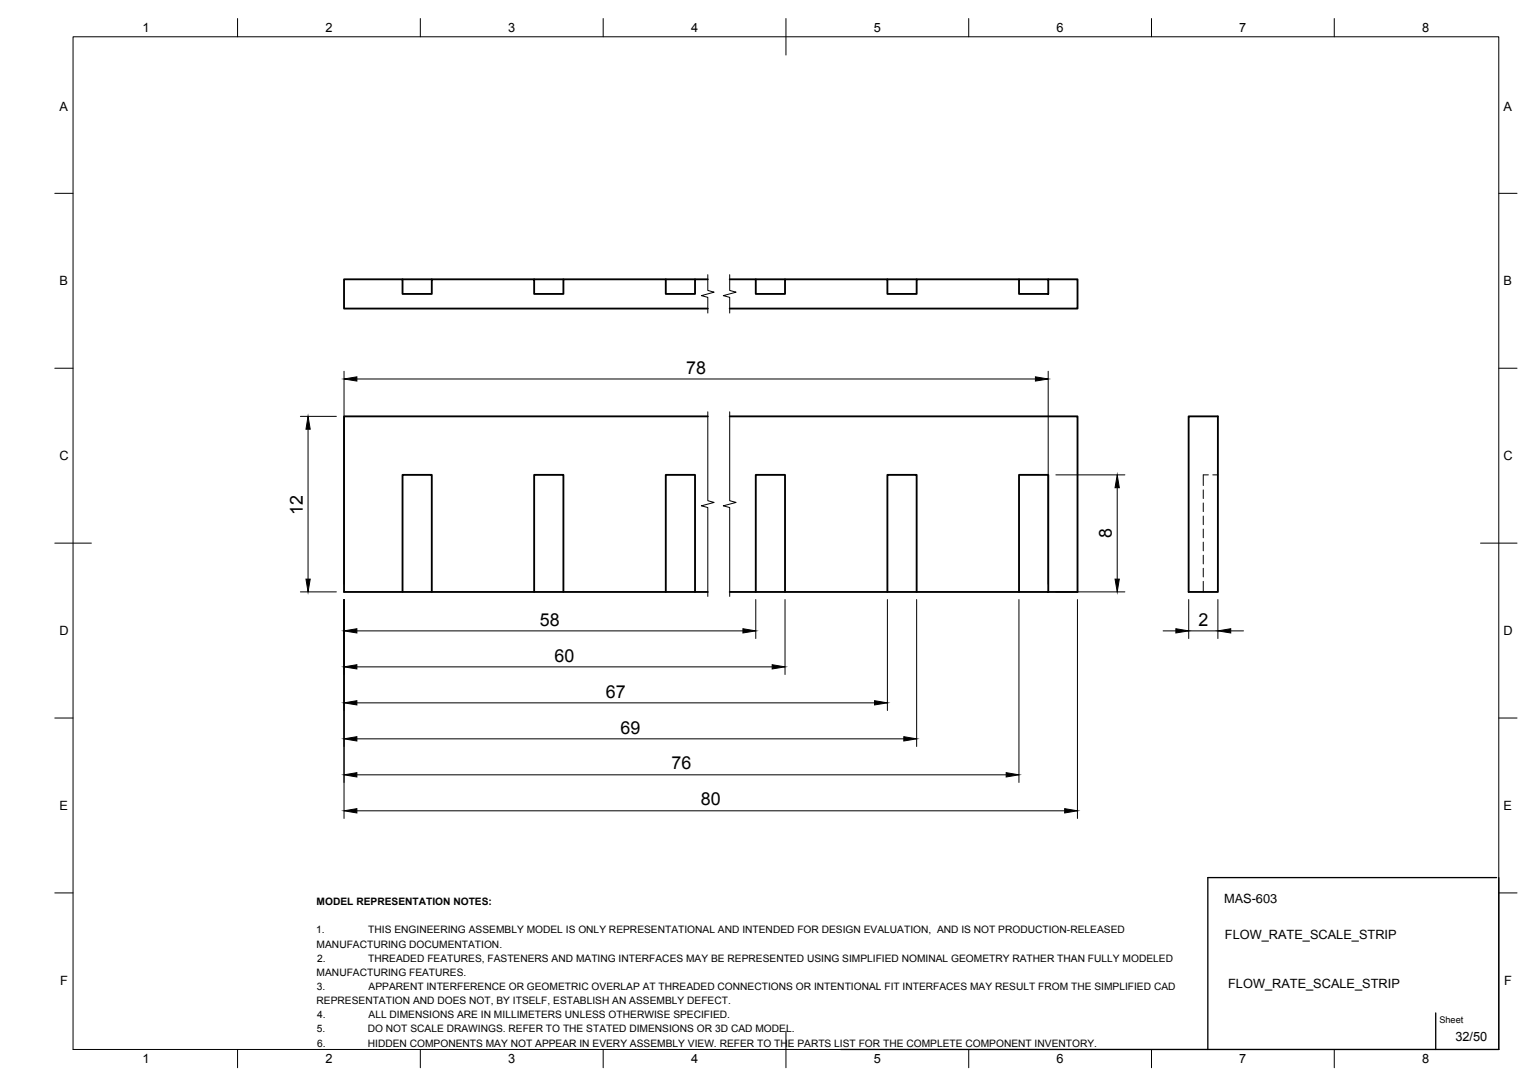
ISO-10303-21;
HEADER;
FILE_DESCRIPTION((''),'2;1');
FILE_NAME('FLOW_RATE_SCALE_STRIP.step','2026-10-01T22:06:14-07:00',(''),(''),'','','');
FILE_SCHEMA (('AUTOMOTIVE_DESIGN { 1 0 10303 214 3 1 1 }'));
ENDSEC;
DATA;
#10=MECHANICAL_DESIGN_GEOMETRIC_PRESENTATION_REPRESENTATION('',(#1004),#50440);
#912=SHAPE_REPRESENTATION_RELATIONSHIP('SRR','None',#50645,#957) ;
#957=ADVANCED_BREP_SHAPE_REPRESENTATION('',(#1059),#50414) ;
#1004=STYLED_ITEM('',(#50886),#1059) ;
#1059=MANIFOLD_SOLID_BREP('FLOW_RATE_SCALE_STRIP',#28671) ;
#2152=PLANE('',#30766) ;
#2153=PLANE('',#30767) ;
#2154=PLANE('',#30768) ;
#2155=PLANE('',#30769) ;
#2156=PLANE('',#30770) ;
#2157=PLANE('',#30771) ;
#2158=PLANE('',#30772) ;
#2159=PLANE('',#30773) ;
#2160=PLANE('',#30774) ;
#2161=PLANE('',#30775) ;
#2162=PLANE('',#30776) ;
#2163=PLANE('',#30777) ;
#2164=PLANE('',#30778) ;
#2165=PLANE('',#30779) ;
#2166=PLANE('',#30780) ;
#2167=PLANE('',#30781) ;
#2168=PLANE('',#30782) ;
#2169=PLANE('',#30783) ;
#2170=PLANE('',#30784) ;
#2171=PLANE('',#30785) ;
#2172=PLANE('',#30786) ;
#2173=PLANE('',#30787) ;
#2174=PLANE('',#30788) ;
#2175=PLANE('',#30789) ;
#2176=PLANE('',#30790) ;
#2177=PLANE('',#30791) ;
#2178=PLANE('',#30792) ;
#2179=PLANE('',#30793) ;
#2180=PLANE('',#30794) ;
#2181=PLANE('',#30795) ;
#2182=PLANE('',#30796) ;
#2183=PLANE('',#30797) ;
#2184=PLANE('',#30798) ;
#2185=PLANE('',#30799) ;
#2186=PLANE('',#30800) ;
#2187=PLANE('',#30801) ;
#2188=PLANE('',#30802) ;
#2189=PLANE('',#30803) ;
#2190=PLANE('',#30804) ;
#2191=PLANE('',#30805) ;
#2192=PLANE('',#30806) ;
#2193=PLANE('',#30807) ;
#3310=FACE_OUTER_BOUND('',#5090,.T.) ;
#3311=FACE_OUTER_BOUND('',#5091,.T.) ;
#3312=FACE_OUTER_BOUND('',#5092,.T.) ;
#3313=FACE_OUTER_BOUND('',#5093,.T.) ;
#3314=FACE_OUTER_BOUND('',#5094,.T.) ;
#3315=FACE_OUTER_BOUND('',#5095,.T.) ;
#3316=FACE_OUTER_BOUND('',#5096,.T.) ;
#3317=FACE_OUTER_BOUND('',#5097,.T.) ;
#3318=FACE_OUTER_BOUND('',#5098,.T.) ;
#3319=FACE_OUTER_BOUND('',#5099,.T.) ;
#3320=FACE_OUTER_BOUND('',#5100,.T.) ;
#3321=FACE_OUTER_BOUND('',#5101,.T.) ;
#3322=FACE_OUTER_BOUND('',#5102,.T.) ;
#3323=FACE_OUTER_BOUND('',#5103,.T.) ;
#3324=FACE_OUTER_BOUND('',#5104,.T.) ;
#3325=FACE_OUTER_BOUND('',#5105,.T.) ;
#3326=FACE_OUTER_BOUND('',#5106,.T.) ;
#3327=FACE_OUTER_BOUND('',#5107,.T.) ;
#3328=FACE_OUTER_BOUND('',#5108,.T.) ;
#3329=FACE_OUTER_BOUND('',#5109,.T.) ;
#3330=FACE_OUTER_BOUND('',#5110,.T.) ;
#3331=FACE_OUTER_BOUND('',#5111,.T.) ;
#3332=FACE_OUTER_BOUND('',#5112,.T.) ;
#3333=FACE_OUTER_BOUND('',#5113,.T.) ;
#3334=FACE_OUTER_BOUND('',#5114,.T.) ;
#3335=FACE_OUTER_BOUND('',#5115,.T.) ;
#3336=FACE_OUTER_BOUND('',#5116,.T.) ;
#3337=FACE_OUTER_BOUND('',#5117,.T.) ;
#3338=FACE_OUTER_BOUND('',#5118,.T.) ;
#3339=FACE_OUTER_BOUND('',#5119,.T.) ;
#3340=FACE_OUTER_BOUND('',#5120,.T.) ;
#3341=FACE_OUTER_BOUND('',#5121,.T.) ;
#3342=FACE_OUTER_BOUND('',#5122,.T.) ;
#3343=FACE_OUTER_BOUND('',#5123,.T.) ;
#3344=FACE_OUTER_BOUND('',#5124,.T.) ;
#3345=FACE_OUTER_BOUND('',#5125,.T.) ;
#3346=FACE_OUTER_BOUND('',#5126,.T.) ;
#3347=FACE_OUTER_BOUND('',#5127,.T.) ;
#3348=FACE_OUTER_BOUND('',#5128,.T.) ;
#3349=FACE_OUTER_BOUND('',#5129,.T.) ;
#3350=FACE_OUTER_BOUND('',#5130,.T.) ;
#3351=FACE_OUTER_BOUND('',#5131,.T.) ;
#5090=EDGE_LOOP('',(#23577,#23578,#23579,#23580)) ;
#5091=EDGE_LOOP('',(#23581,#23582,#23583,#23584)) ;
#5092=EDGE_LOOP('',(#23585,#23586,#23587,#23588)) ;
#5093=EDGE_LOOP('',(#23589,#23590,#23591,#23592)) ;
#5094=EDGE_LOOP('',(#23593,#23594,#23595,#23596,#23597,#23598,#23599,#23600,
#23601,#23602,#23603,#23604,#23605,#23606,#23607,#23608,#23609,#23610,#23611,
#23612,#23613,#23614,#23615,#23616,#23617,#23618,#23619,#23620,#23621,#23622,
#23623,#23624,#23625,#23626,#23627,#23628,#23629,#23630,#23631,#23632)) ;
#5095=EDGE_LOOP('',(#23633,#23634,#23635,#23636)) ;
#5096=EDGE_LOOP('',(#23637,#23638,#23639,#23640)) ;
#5097=EDGE_LOOP('',(#23641,#23642,#23643,#23644)) ;
#5098=EDGE_LOOP('',(#23645,#23646,#23647,#23648)) ;
#5099=EDGE_LOOP('',(#23649,#23650,#23651,#23652,#23653,#23654,#23655,#23656,
#23657,#23658,#23659,#23660,#23661,#23662,#23663,#23664,#23665,#23666,#23667,
#23668,#23669,#23670,#23671,#23672,#23673,#23674,#23675,#23676,#23677,#23678,
#23679,#23680,#23681,#23682,#23683,#23684,#23685,#23686,#23687,#23688)) ;
#5100=EDGE_LOOP('',(#23689,#23690,#23691,#23692)) ;
#5101=EDGE_LOOP('',(#23693,#23694,#23695,#23696)) ;
#5102=EDGE_LOOP('',(#23697,#23698,#23699,#23700)) ;
#5103=EDGE_LOOP('',(#23701,#23702,#23703,#23704)) ;
#5104=EDGE_LOOP('',(#23705,#23706,#23707,#23708)) ;
#5105=EDGE_LOOP('',(#23709,#23710,#23711,#23712)) ;
#5106=EDGE_LOOP('',(#23713,#23714,#23715,#23716)) ;
#5107=EDGE_LOOP('',(#23717,#23718,#23719,#23720)) ;
#5108=EDGE_LOOP('',(#23721,#23722,#23723,#23724)) ;
#5109=EDGE_LOOP('',(#23725,#23726,#23727,#23728)) ;
#5110=EDGE_LOOP('',(#23729,#23730,#23731,#23732)) ;
#5111=EDGE_LOOP('',(#23733,#23734,#23735,#23736)) ;
#5112=EDGE_LOOP('',(#23737,#23738,#23739,#23740)) ;
#5113=EDGE_LOOP('',(#23741,#23742,#23743,#23744)) ;
#5114=EDGE_LOOP('',(#23745,#23746,#23747,#23748)) ;
#5115=EDGE_LOOP('',(#23749,#23750,#23751,#23752)) ;
#5116=EDGE_LOOP('',(#23753,#23754,#23755,#23756)) ;
#5117=EDGE_LOOP('',(#23757,#23758,#23759,#23760)) ;
#5118=EDGE_LOOP('',(#23761,#23762,#23763,#23764)) ;
#5119=EDGE_LOOP('',(#23765,#23766,#23767,#23768)) ;
#5120=EDGE_LOOP('',(#23769,#23770,#23771,#23772)) ;
#5121=EDGE_LOOP('',(#23773,#23774,#23775,#23776)) ;
#5122=EDGE_LOOP('',(#23777,#23778,#23779,#23780)) ;
#5123=EDGE_LOOP('',(#23781,#23782,#23783,#23784)) ;
#5124=EDGE_LOOP('',(#23785,#23786,#23787,#23788)) ;
#5125=EDGE_LOOP('',(#23789,#23790,#23791,#23792)) ;
#5126=EDGE_LOOP('',(#23793,#23794,#23795,#23796)) ;
#5127=EDGE_LOOP('',(#23797,#23798,#23799,#23800)) ;
#5128=EDGE_LOOP('',(#23801,#23802,#23803,#23804)) ;
#5129=EDGE_LOOP('',(#23805,#23806,#23807,#23808)) ;
#5130=EDGE_LOOP('',(#23809,#23810,#23811,#23812)) ;
#5131=EDGE_LOOP('',(#23813,#23814,#23815,#23816)) ;
#7679=LINE('',#46561,#10151) ;
#7680=LINE('',#46563,#10152) ;
#7681=LINE('',#46565,#10153) ;
#7682=LINE('',#46566,#10154) ;
#7683=LINE('',#46569,#10155) ;
#7684=LINE('',#46571,#10156) ;
#7685=LINE('',#46572,#10157) ;
#7686=LINE('',#46575,#10158) ;
#7687=LINE('',#46576,#10159) ;
#7688=LINE('',#46579,#10160) ;
#7689=LINE('',#46580,#10161) ;
#7690=LINE('',#46583,#10162) ;
#7691=LINE('',#46585,#10163) ;
#7692=LINE('',#46587,#10164) ;
#7693=LINE('',#46589,#10165) ;
#7694=LINE('',#46591,#10166) ;
#7695=LINE('',#46593,#10167) ;
#7696=LINE('',#46595,#10168) ;
#7697=LINE('',#46597,#10169) ;
#7698=LINE('',#46599,#10170) ;
#7699=LINE('',#46601,#10171) ;
#7700=LINE('',#46603,#10172) ;
#7701=LINE('',#46605,#10173) ;
#7702=LINE('',#46607,#10174) ;
#7703=LINE('',#46609,#10175) ;
#7704=LINE('',#46611,#10176) ;
#7705=LINE('',#46613,#10177) ;
#7706=LINE('',#46615,#10178) ;
#7707=LINE('',#46617,#10179) ;
#7708=LINE('',#46619,#10180) ;
#7709=LINE('',#46621,#10181) ;
#7710=LINE('',#46623,#10182) ;
#7711=LINE('',#46625,#10183) ;
#7712=LINE('',#46627,#10184) ;
#7713=LINE('',#46629,#10185) ;
#7714=LINE('',#46631,#10186) ;
#7715=LINE('',#46633,#10187) ;
#7716=LINE('',#46635,#10188) ;
#7717=LINE('',#46637,#10189) ;
#7718=LINE('',#46639,#10190) ;
#7719=LINE('',#46641,#10191) ;
#7720=LINE('',#46643,#10192) ;
#7721=LINE('',#46645,#10193) ;
#7722=LINE('',#46647,#10194) ;
#7723=LINE('',#46649,#10195) ;
#7724=LINE('',#46651,#10196) ;
#7725=LINE('',#46653,#10197) ;
#7726=LINE('',#46654,#10198) ;
#7727=LINE('',#46658,#10199) ;
#7728=LINE('',#46660,#10200) ;
#7729=LINE('',#46662,#10201) ;
#7730=LINE('',#46663,#10202) ;
#7731=LINE('',#46665,#10203) ;
#7732=LINE('',#46666,#10204) ;
#7733=LINE('',#46668,#10205) ;
#7734=LINE('',#46670,#10206) ;
#7735=LINE('',#46673,#10207) ;
#7736=LINE('',#46675,#10208) ;
#7737=LINE('',#46676,#10209) ;
#7738=LINE('',#46678,#10210) ;
#7739=LINE('',#46680,#10211) ;
#7740=LINE('',#46681,#10212) ;
#7741=LINE('',#46683,#10213) ;
#7742=LINE('',#46685,#10214) ;
#7743=LINE('',#46686,#10215) ;
#7744=LINE('',#46688,#10216) ;
#7745=LINE('',#46690,#10217) ;
#7746=LINE('',#46691,#10218) ;
#7747=LINE('',#46693,#10219) ;
#7748=LINE('',#46695,#10220) ;
#7749=LINE('',#46696,#10221) ;
#7750=LINE('',#46698,#10222) ;
#7751=LINE('',#46700,#10223) ;
#7752=LINE('',#46701,#10224) ;
#7753=LINE('',#46703,#10225) ;
#7754=LINE('',#46705,#10226) ;
#7755=LINE('',#46706,#10227) ;
#7756=LINE('',#46708,#10228) ;
#7757=LINE('',#46710,#10229) ;
#7758=LINE('',#46711,#10230) ;
#7759=LINE('',#46714,#10231) ;
#7760=LINE('',#46716,#10232) ;
#7761=LINE('',#46717,#10233) ;
#7762=LINE('',#46719,#10234) ;
#7763=LINE('',#46721,#10235) ;
#7764=LINE('',#46725,#10236) ;
#7765=LINE('',#46727,#10237) ;
#7766=LINE('',#46728,#10238) ;
#7767=LINE('',#46730,#10239) ;
#7768=LINE('',#46732,#10240) ;
#7769=LINE('',#46736,#10241) ;
#7770=LINE('',#46738,#10242) ;
#7771=LINE('',#46739,#10243) ;
#7772=LINE('',#46741,#10244) ;
#7773=LINE('',#46743,#10245) ;
#7774=LINE('',#46747,#10246) ;
#7775=LINE('',#46749,#10247) ;
#7776=LINE('',#46750,#10248) ;
#7777=LINE('',#46752,#10249) ;
#7778=LINE('',#46754,#10250) ;
#7779=LINE('',#46758,#10251) ;
#7780=LINE('',#46760,#10252) ;
#7781=LINE('',#46761,#10253) ;
#7782=LINE('',#46763,#10254) ;
#7783=LINE('',#46765,#10255) ;
#7784=LINE('',#46769,#10256) ;
#7785=LINE('',#46771,#10257) ;
#7786=LINE('',#46772,#10258) ;
#7787=LINE('',#46774,#10259) ;
#7788=LINE('',#46776,#10260) ;
#7789=LINE('',#46780,#10261) ;
#7790=LINE('',#46782,#10262) ;
#7791=LINE('',#46783,#10263) ;
#7792=LINE('',#46785,#10264) ;
#7793=LINE('',#46787,#10265) ;
#7794=LINE('',#46791,#10266) ;
#7795=LINE('',#46793,#10267) ;
#7796=LINE('',#46794,#10268) ;
#7797=LINE('',#46796,#10269) ;
#7798=LINE('',#46798,#10270) ;
#10151=VECTOR('',#37438,1.) ;
#10152=VECTOR('',#37439,1.) ;
#10153=VECTOR('',#37440,1.) ;
#10154=VECTOR('',#37441,1.) ;
#10155=VECTOR('',#37444,1.) ;
#10156=VECTOR('',#37445,1.) ;
#10157=VECTOR('',#37446,1.) ;
#10158=VECTOR('',#37449,1.) ;
#10159=VECTOR('',#37450,1.) ;
#10160=VECTOR('',#37453,1.) ;
#10161=VECTOR('',#37454,1.) ;
#10162=VECTOR('',#37457,1.) ;
#10163=VECTOR('',#37458,1.) ;
#10164=VECTOR('',#37459,1.) ;
#10165=VECTOR('',#37460,1.) ;
#10166=VECTOR('',#37461,1.) ;
#10167=VECTOR('',#37462,1.) ;
#10168=VECTOR('',#37463,1.) ;
#10169=VECTOR('',#37464,1.) ;
#10170=VECTOR('',#37465,1.) ;
#10171=VECTOR('',#37466,1.) ;
#10172=VECTOR('',#37467,1.) ;
#10173=VECTOR('',#37468,1.) ;
#10174=VECTOR('',#37469,1.) ;
#10175=VECTOR('',#37470,1.) ;
#10176=VECTOR('',#37471,1.) ;
#10177=VECTOR('',#37472,1.) ;
#10178=VECTOR('',#37473,1.) ;
#10179=VECTOR('',#37474,1.) ;
#10180=VECTOR('',#37475,1.) ;
#10181=VECTOR('',#37476,1.) ;
#10182=VECTOR('',#37477,1.) ;
#10183=VECTOR('',#37478,1.) ;
#10184=VECTOR('',#37479,1.) ;
#10185=VECTOR('',#37480,1.) ;
#10186=VECTOR('',#37481,1.) ;
#10187=VECTOR('',#37482,1.) ;
#10188=VECTOR('',#37483,1.) ;
#10189=VECTOR('',#37484,1.) ;
#10190=VECTOR('',#37485,1.) ;
#10191=VECTOR('',#37486,1.) ;
#10192=VECTOR('',#37487,1.) ;
#10193=VECTOR('',#37488,1.) ;
#10194=VECTOR('',#37489,1.) ;
#10195=VECTOR('',#37490,1.) ;
#10196=VECTOR('',#37491,1.) ;
#10197=VECTOR('',#37492,1.) ;
#10198=VECTOR('',#37493,1.) ;
#10199=VECTOR('',#37496,1.) ;
#10200=VECTOR('',#37497,1.) ;
#10201=VECTOR('',#37498,1.) ;
#10202=VECTOR('',#37499,1.) ;
#10203=VECTOR('',#37502,1.) ;
#10204=VECTOR('',#37503,1.) ;
#10205=VECTOR('',#37506,1.) ;
#10206=VECTOR('',#37509,1.) ;
#10207=VECTOR('',#37512,1.) ;
#10208=VECTOR('',#37513,1.) ;
#10209=VECTOR('',#37514,1.) ;
#10210=VECTOR('',#37515,1.) ;
#10211=VECTOR('',#37516,1.) ;
#10212=VECTOR('',#37517,1.) ;
#10213=VECTOR('',#37518,1.) ;
#10214=VECTOR('',#37519,1.) ;
#10215=VECTOR('',#37520,1.) ;
#10216=VECTOR('',#37521,1.) ;
#10217=VECTOR('',#37522,1.) ;
#10218=VECTOR('',#37523,1.) ;
#10219=VECTOR('',#37524,1.) ;
#10220=VECTOR('',#37525,1.) ;
#10221=VECTOR('',#37526,1.) ;
#10222=VECTOR('',#37527,1.) ;
#10223=VECTOR('',#37528,1.) ;
#10224=VECTOR('',#37529,1.) ;
#10225=VECTOR('',#37530,1.) ;
#10226=VECTOR('',#37531,1.) ;
#10227=VECTOR('',#37532,1.) ;
#10228=VECTOR('',#37533,1.) ;
#10229=VECTOR('',#37534,1.) ;
#10230=VECTOR('',#37535,1.) ;
#10231=VECTOR('',#37538,1.) ;
#10232=VECTOR('',#37539,1.) ;
#10233=VECTOR('',#37540,1.) ;
#10234=VECTOR('',#37543,1.) ;
#10235=VECTOR('',#37546,1.) ;
#10236=VECTOR('',#37551,1.) ;
#10237=VECTOR('',#37552,1.) ;
#10238=VECTOR('',#37553,1.) ;
#10239=VECTOR('',#37556,1.) ;
#10240=VECTOR('',#37559,1.) ;
#10241=VECTOR('',#37564,1.) ;
#10242=VECTOR('',#37565,1.) ;
#10243=VECTOR('',#37566,1.) ;
#10244=VECTOR('',#37569,1.) ;
#10245=VECTOR('',#37572,1.) ;
#10246=VECTOR('',#37577,1.) ;
#10247=VECTOR('',#37578,1.) ;
#10248=VECTOR('',#37579,1.) ;
#10249=VECTOR('',#37582,1.) ;
#10250=VECTOR('',#37585,1.) ;
#10251=VECTOR('',#37590,1.) ;
#10252=VECTOR('',#37591,1.) ;
#10253=VECTOR('',#37592,1.) ;
#10254=VECTOR('',#37595,1.) ;
#10255=VECTOR('',#37598,1.) ;
#10256=VECTOR('',#37603,1.) ;
#10257=VECTOR('',#37604,1.) ;
#10258=VECTOR('',#37605,1.) ;
#10259=VECTOR('',#37608,1.) ;
#10260=VECTOR('',#37611,1.) ;
#10261=VECTOR('',#37616,1.) ;
#10262=VECTOR('',#37617,1.) ;
#10263=VECTOR('',#37618,1.) ;
#10264=VECTOR('',#37621,1.) ;
#10265=VECTOR('',#37624,1.) ;
#10266=VECTOR('',#37629,1.) ;
#10267=VECTOR('',#37630,1.) ;
#10268=VECTOR('',#37631,1.) ;
#10269=VECTOR('',#37634,1.) ;
#10270=VECTOR('',#37637,1.) ;
#13508=VERTEX_POINT('',#46559) ;
#13509=VERTEX_POINT('',#46560) ;
#13510=VERTEX_POINT('',#46562) ;
#13511=VERTEX_POINT('',#46564) ;
#13512=VERTEX_POINT('',#46568) ;
#13513=VERTEX_POINT('',#46570) ;
#13514=VERTEX_POINT('',#46574) ;
#13515=VERTEX_POINT('',#46578) ;
#13516=VERTEX_POINT('',#46582) ;
#13517=VERTEX_POINT('',#46584) ;
#13518=VERTEX_POINT('',#46586) ;
#13519=VERTEX_POINT('',#46588) ;
#13520=VERTEX_POINT('',#46590) ;
#13521=VERTEX_POINT('',#46592) ;
#13522=VERTEX_POINT('',#46594) ;
#13523=VERTEX_POINT('',#46596) ;
#13524=VERTEX_POINT('',#46598) ;
#13525=VERTEX_POINT('',#46600) ;
#13526=VERTEX_POINT('',#46602) ;
#13527=VERTEX_POINT('',#46604) ;
#13528=VERTEX_POINT('',#46606) ;
#13529=VERTEX_POINT('',#46608) ;
#13530=VERTEX_POINT('',#46610) ;
#13531=VERTEX_POINT('',#46612) ;
#13532=VERTEX_POINT('',#46614) ;
#13533=VERTEX_POINT('',#46616) ;
#13534=VERTEX_POINT('',#46618) ;
#13535=VERTEX_POINT('',#46620) ;
#13536=VERTEX_POINT('',#46622) ;
#13537=VERTEX_POINT('',#46624) ;
#13538=VERTEX_POINT('',#46626) ;
#13539=VERTEX_POINT('',#46628) ;
#13540=VERTEX_POINT('',#46630) ;
#13541=VERTEX_POINT('',#46632) ;
#13542=VERTEX_POINT('',#46634) ;
#13543=VERTEX_POINT('',#46636) ;
#13544=VERTEX_POINT('',#46638) ;
#13545=VERTEX_POINT('',#46640) ;
#13546=VERTEX_POINT('',#46642) ;
#13547=VERTEX_POINT('',#46644) ;
#13548=VERTEX_POINT('',#46646) ;
#13549=VERTEX_POINT('',#46648) ;
#13550=VERTEX_POINT('',#46650) ;
#13551=VERTEX_POINT('',#46652) ;
#13552=VERTEX_POINT('',#46656) ;
#13553=VERTEX_POINT('',#46657) ;
#13554=VERTEX_POINT('',#46659) ;
#13555=VERTEX_POINT('',#46661) ;
#13556=VERTEX_POINT('',#46672) ;
#13557=VERTEX_POINT('',#46674) ;
#13558=VERTEX_POINT('',#46677) ;
#13559=VERTEX_POINT('',#46679) ;
#13560=VERTEX_POINT('',#46682) ;
#13561=VERTEX_POINT('',#46684) ;
#13562=VERTEX_POINT('',#46687) ;
#13563=VERTEX_POINT('',#46689) ;
#13564=VERTEX_POINT('',#46692) ;
#13565=VERTEX_POINT('',#46694) ;
#13566=VERTEX_POINT('',#46697) ;
#13567=VERTEX_POINT('',#46699) ;
#13568=VERTEX_POINT('',#46702) ;
#13569=VERTEX_POINT('',#46704) ;
#13570=VERTEX_POINT('',#46707) ;
#13571=VERTEX_POINT('',#46709) ;
#13572=VERTEX_POINT('',#46713) ;
#13573=VERTEX_POINT('',#46715) ;
#13574=VERTEX_POINT('',#46724) ;
#13575=VERTEX_POINT('',#46726) ;
#13576=VERTEX_POINT('',#46735) ;
#13577=VERTEX_POINT('',#46737) ;
#13578=VERTEX_POINT('',#46746) ;
#13579=VERTEX_POINT('',#46748) ;
#13580=VERTEX_POINT('',#46757) ;
#13581=VERTEX_POINT('',#46759) ;
#13582=VERTEX_POINT('',#46768) ;
#13583=VERTEX_POINT('',#46770) ;
#13584=VERTEX_POINT('',#46779) ;
#13585=VERTEX_POINT('',#46781) ;
#13586=VERTEX_POINT('',#46790) ;
#13587=VERTEX_POINT('',#46792) ;
#17054=EDGE_CURVE('',#13508,#13509,#7679,.T.) ;
#17055=EDGE_CURVE('',#13510,#13508,#7680,.T.) ;
#17056=EDGE_CURVE('',#13511,#13510,#7681,.T.) ;
#17057=EDGE_CURVE('',#13509,#13511,#7682,.T.) ;
#17058=EDGE_CURVE('',#13509,#13512,#7683,.T.) ;
#17059=EDGE_CURVE('',#13513,#13511,#7684,.T.) ;
#17060=EDGE_CURVE('',#13512,#13513,#7685,.T.) ;
#17061=EDGE_CURVE('',#13513,#13514,#7686,.T.) ;
#17062=EDGE_CURVE('',#13514,#13510,#7687,.T.) ;
#17063=EDGE_CURVE('',#13515,#13508,#7688,.T.) ;
#17064=EDGE_CURVE('',#13514,#13515,#7689,.T.) ;
#17065=EDGE_CURVE('',#13516,#13512,#7690,.T.) ;
#17066=EDGE_CURVE('',#13516,#13517,#7691,.T.) ;
#17067=EDGE_CURVE('',#13517,#13518,#7692,.T.) ;
#17068=EDGE_CURVE('',#13518,#13519,#7693,.T.) ;
#17069=EDGE_CURVE('',#13520,#13519,#7694,.T.) ;
#17070=EDGE_CURVE('',#13520,#13521,#7695,.T.) ;
#17071=EDGE_CURVE('',#13521,#13522,#7696,.T.) ;
#17072=EDGE_CURVE('',#13522,#13523,#7697,.T.) ;
#17073=EDGE_CURVE('',#13524,#13523,#7698,.T.) ;
#17074=EDGE_CURVE('',#13524,#13525,#7699,.T.) ;
#17075=EDGE_CURVE('',#13525,#13526,#7700,.T.) ;
#17076=EDGE_CURVE('',#13526,#13527,#7701,.T.) ;
#17077=EDGE_CURVE('',#13528,#13527,#7702,.T.) ;
#17078=EDGE_CURVE('',#13528,#13529,#7703,.T.) ;
#17079=EDGE_CURVE('',#13529,#13530,#7704,.T.) ;
#17080=EDGE_CURVE('',#13530,#13531,#7705,.T.) ;
#17081=EDGE_CURVE('',#13532,#13531,#7706,.T.) ;
#17082=EDGE_CURVE('',#13532,#13533,#7707,.T.) ;
#17083=EDGE_CURVE('',#13533,#13534,#7708,.T.) ;
#17084=EDGE_CURVE('',#13534,#13535,#7709,.T.) ;
#17085=EDGE_CURVE('',#13536,#13535,#7710,.T.) ;
#17086=EDGE_CURVE('',#13536,#13537,#7711,.T.) ;
#17087=EDGE_CURVE('',#13537,#13538,#7712,.T.) ;
#17088=EDGE_CURVE('',#13538,#13539,#7713,.T.) ;
#17089=EDGE_CURVE('',#13540,#13539,#7714,.T.) ;
#17090=EDGE_CURVE('',#13540,#13541,#7715,.T.) ;
#17091=EDGE_CURVE('',#13541,#13542,#7716,.T.) ;
#17092=EDGE_CURVE('',#13542,#13543,#7717,.T.) ;
#17093=EDGE_CURVE('',#13544,#13543,#7718,.T.) ;
#17094=EDGE_CURVE('',#13544,#13545,#7719,.T.) ;
#17095=EDGE_CURVE('',#13545,#13546,#7720,.T.) ;
#17096=EDGE_CURVE('',#13546,#13547,#7721,.T.) ;
#17097=EDGE_CURVE('',#13548,#13547,#7722,.T.) ;
#17098=EDGE_CURVE('',#13548,#13549,#7723,.T.) ;
#17099=EDGE_CURVE('',#13550,#13549,#7724,.T.) ;
#17100=EDGE_CURVE('',#13551,#13550,#7725,.T.) ;
#17101=EDGE_CURVE('',#13515,#13551,#7726,.T.) ;
#17102=EDGE_CURVE('',#13552,#13553,#7727,.T.) ;
#17103=EDGE_CURVE('',#13552,#13554,#7728,.T.) ;
#17104=EDGE_CURVE('',#13554,#13555,#7729,.T.) ;
#17105=EDGE_CURVE('',#13553,#13555,#7730,.T.) ;
#17106=EDGE_CURVE('',#13553,#13516,#7731,.T.) ;
#17107=EDGE_CURVE('',#13555,#13517,#7732,.T.) ;
#17108=EDGE_CURVE('',#13518,#13554,#7733,.T.) ;
#17109=EDGE_CURVE('',#13519,#13552,#7734,.T.) ;
#17110=EDGE_CURVE('',#13551,#13556,#7735,.T.) ;
#17111=EDGE_CURVE('',#13556,#13557,#7736,.T.) ;
#17112=EDGE_CURVE('',#13557,#13548,#7737,.T.) ;
#17113=EDGE_CURVE('',#13547,#13558,#7738,.T.) ;
#17114=EDGE_CURVE('',#13558,#13559,#7739,.T.) ;
#17115=EDGE_CURVE('',#13559,#13544,#7740,.T.) ;
#17116=EDGE_CURVE('',#13543,#13560,#7741,.T.) ;
#17117=EDGE_CURVE('',#13560,#13561,#7742,.T.) ;
#17118=EDGE_CURVE('',#13561,#13540,#7743,.T.) ;
#17119=EDGE_CURVE('',#13539,#13562,#7744,.T.) ;
#17120=EDGE_CURVE('',#13562,#13563,#7745,.T.) ;
#17121=EDGE_CURVE('',#13563,#13536,#7746,.T.) ;
#17122=EDGE_CURVE('',#13535,#13564,#7747,.T.) ;
#17123=EDGE_CURVE('',#13564,#13565,#7748,.T.) ;
#17124=EDGE_CURVE('',#13565,#13532,#7749,.T.) ;
#17125=EDGE_CURVE('',#13531,#13566,#7750,.T.) ;
#17126=EDGE_CURVE('',#13566,#13567,#7751,.T.) ;
#17127=EDGE_CURVE('',#13567,#13528,#7752,.T.) ;
#17128=EDGE_CURVE('',#13527,#13568,#7753,.T.) ;
#17129=EDGE_CURVE('',#13568,#13569,#7754,.T.) ;
#17130=EDGE_CURVE('',#13569,#13524,#7755,.T.) ;
#17131=EDGE_CURVE('',#13523,#13570,#7756,.T.) ;
#17132=EDGE_CURVE('',#13570,#13571,#7757,.T.) ;
#17133=EDGE_CURVE('',#13571,#13520,#7758,.T.) ;
#17134=EDGE_CURVE('',#13572,#13521,#7759,.T.) ;
#17135=EDGE_CURVE('',#13573,#13572,#7760,.T.) ;
#17136=EDGE_CURVE('',#13522,#13573,#7761,.T.) ;
#17137=EDGE_CURVE('',#13570,#13573,#7762,.T.) ;
#17138=EDGE_CURVE('',#13571,#13572,#7763,.T.) ;
#17139=EDGE_CURVE('',#13568,#13574,#7764,.T.) ;
#17140=EDGE_CURVE('',#13574,#13575,#7765,.T.) ;
#17141=EDGE_CURVE('',#13569,#13575,#7766,.T.) ;
#17142=EDGE_CURVE('',#13575,#13525,#7767,.T.) ;
#17143=EDGE_CURVE('',#13526,#13574,#7768,.T.) ;
#17144=EDGE_CURVE('',#13576,#13529,#7769,.T.) ;
#17145=EDGE_CURVE('',#13577,#13576,#7770,.T.) ;
#17146=EDGE_CURVE('',#13530,#13577,#7771,.T.) ;
#17147=EDGE_CURVE('',#13566,#13577,#7772,.T.) ;
#17148=EDGE_CURVE('',#13567,#13576,#7773,.T.) ;
#17149=EDGE_CURVE('',#13564,#13578,#7774,.T.) ;
#17150=EDGE_CURVE('',#13578,#13579,#7775,.T.) ;
#17151=EDGE_CURVE('',#13565,#13579,#7776,.T.) ;
#17152=EDGE_CURVE('',#13579,#13533,#7777,.T.) ;
#17153=EDGE_CURVE('',#13534,#13578,#7778,.T.) ;
#17154=EDGE_CURVE('',#13580,#13537,#7779,.T.) ;
#17155=EDGE_CURVE('',#13581,#13580,#7780,.T.) ;
#17156=EDGE_CURVE('',#13538,#13581,#7781,.T.) ;
#17157=EDGE_CURVE('',#13562,#13581,#7782,.T.) ;
#17158=EDGE_CURVE('',#13563,#13580,#7783,.T.) ;
#17159=EDGE_CURVE('',#13560,#13582,#7784,.T.) ;
#17160=EDGE_CURVE('',#13582,#13583,#7785,.T.) ;
#17161=EDGE_CURVE('',#13561,#13583,#7786,.T.) ;
#17162=EDGE_CURVE('',#13583,#13541,#7787,.T.) ;
#17163=EDGE_CURVE('',#13542,#13582,#7788,.T.) ;
#17164=EDGE_CURVE('',#13584,#13545,#7789,.T.) ;
#17165=EDGE_CURVE('',#13585,#13584,#7790,.T.) ;
#17166=EDGE_CURVE('',#13546,#13585,#7791,.T.) ;
#17167=EDGE_CURVE('',#13558,#13585,#7792,.T.) ;
#17168=EDGE_CURVE('',#13559,#13584,#7793,.T.) ;
#17169=EDGE_CURVE('',#13586,#13550,#7794,.T.) ;
#17170=EDGE_CURVE('',#13549,#13587,#7795,.T.) ;
#17171=EDGE_CURVE('',#13587,#13586,#7796,.T.) ;
#17172=EDGE_CURVE('',#13557,#13587,#7797,.T.) ;
#17173=EDGE_CURVE('',#13556,#13586,#7798,.T.) ;
#23577=ORIENTED_EDGE('',*,*,#17054,.F.) ;
#23578=ORIENTED_EDGE('',*,*,#17055,.F.) ;
#23579=ORIENTED_EDGE('',*,*,#17056,.F.) ;
#23580=ORIENTED_EDGE('',*,*,#17057,.F.) ;
#23581=ORIENTED_EDGE('',*,*,#17058,.F.) ;
#23582=ORIENTED_EDGE('',*,*,#17057,.T.) ;
#23583=ORIENTED_EDGE('',*,*,#17059,.F.) ;
#23584=ORIENTED_EDGE('',*,*,#17060,.F.) ;
#23585=ORIENTED_EDGE('',*,*,#17061,.F.) ;
#23586=ORIENTED_EDGE('',*,*,#17059,.T.) ;
#23587=ORIENTED_EDGE('',*,*,#17056,.T.) ;
#23588=ORIENTED_EDGE('',*,*,#17062,.F.) ;
#23589=ORIENTED_EDGE('',*,*,#17063,.F.) ;
#23590=ORIENTED_EDGE('',*,*,#17064,.F.) ;
#23591=ORIENTED_EDGE('',*,*,#17062,.T.) ;
#23592=ORIENTED_EDGE('',*,*,#17055,.T.) ;
#23593=ORIENTED_EDGE('',*,*,#17063,.T.) ;
#23594=ORIENTED_EDGE('',*,*,#17054,.T.) ;
#23595=ORIENTED_EDGE('',*,*,#17058,.T.) ;
#23596=ORIENTED_EDGE('',*,*,#17065,.F.) ;
#23597=ORIENTED_EDGE('',*,*,#17066,.T.) ;
#23598=ORIENTED_EDGE('',*,*,#17067,.T.) ;
#23599=ORIENTED_EDGE('',*,*,#17068,.T.) ;
#23600=ORIENTED_EDGE('',*,*,#17069,.F.) ;
#23601=ORIENTED_EDGE('',*,*,#17070,.T.) ;
#23602=ORIENTED_EDGE('',*,*,#17071,.T.) ;
#23603=ORIENTED_EDGE('',*,*,#17072,.T.) ;
#23604=ORIENTED_EDGE('',*,*,#17073,.F.) ;
#23605=ORIENTED_EDGE('',*,*,#17074,.T.) ;
#23606=ORIENTED_EDGE('',*,*,#17075,.T.) ;
#23607=ORIENTED_EDGE('',*,*,#17076,.T.) ;
#23608=ORIENTED_EDGE('',*,*,#17077,.F.) ;
#23609=ORIENTED_EDGE('',*,*,#17078,.T.) ;
#23610=ORIENTED_EDGE('',*,*,#17079,.T.) ;
#23611=ORIENTED_EDGE('',*,*,#17080,.T.) ;
#23612=ORIENTED_EDGE('',*,*,#17081,.F.) ;
#23613=ORIENTED_EDGE('',*,*,#17082,.T.) ;
#23614=ORIENTED_EDGE('',*,*,#17083,.T.) ;
#23615=ORIENTED_EDGE('',*,*,#17084,.T.) ;
#23616=ORIENTED_EDGE('',*,*,#17085,.F.) ;
#23617=ORIENTED_EDGE('',*,*,#17086,.T.) ;
#23618=ORIENTED_EDGE('',*,*,#17087,.T.) ;
#23619=ORIENTED_EDGE('',*,*,#17088,.T.) ;
#23620=ORIENTED_EDGE('',*,*,#17089,.F.) ;
#23621=ORIENTED_EDGE('',*,*,#17090,.T.) ;
#23622=ORIENTED_EDGE('',*,*,#17091,.T.) ;
#23623=ORIENTED_EDGE('',*,*,#17092,.T.) ;
#23624=ORIENTED_EDGE('',*,*,#17093,.F.) ;
#23625=ORIENTED_EDGE('',*,*,#17094,.T.) ;
#23626=ORIENTED_EDGE('',*,*,#17095,.T.) ;
#23627=ORIENTED_EDGE('',*,*,#17096,.T.) ;
#23628=ORIENTED_EDGE('',*,*,#17097,.F.) ;
#23629=ORIENTED_EDGE('',*,*,#17098,.T.) ;
#23630=ORIENTED_EDGE('',*,*,#17099,.F.) ;
#23631=ORIENTED_EDGE('',*,*,#17100,.F.) ;
#23632=ORIENTED_EDGE('',*,*,#17101,.F.) ;
#23633=ORIENTED_EDGE('',*,*,#17102,.F.) ;
#23634=ORIENTED_EDGE('',*,*,#17103,.T.) ;
#23635=ORIENTED_EDGE('',*,*,#17104,.T.) ;
#23636=ORIENTED_EDGE('',*,*,#17105,.F.) ;
#23637=ORIENTED_EDGE('',*,*,#17106,.F.) ;
#23638=ORIENTED_EDGE('',*,*,#17105,.T.) ;
#23639=ORIENTED_EDGE('',*,*,#17107,.T.) ;
#23640=ORIENTED_EDGE('',*,*,#17066,.F.) ;
#23641=ORIENTED_EDGE('',*,*,#17067,.F.) ;
#23642=ORIENTED_EDGE('',*,*,#17107,.F.) ;
#23643=ORIENTED_EDGE('',*,*,#17104,.F.) ;
#23644=ORIENTED_EDGE('',*,*,#17108,.F.) ;
#23645=ORIENTED_EDGE('',*,*,#17109,.F.) ;
#23646=ORIENTED_EDGE('',*,*,#17068,.F.) ;
#23647=ORIENTED_EDGE('',*,*,#17108,.T.) ;
#23648=ORIENTED_EDGE('',*,*,#17103,.F.) ;
#23649=ORIENTED_EDGE('',*,*,#17064,.T.) ;
#23650=ORIENTED_EDGE('',*,*,#17101,.T.) ;
#23651=ORIENTED_EDGE('',*,*,#17110,.T.) ;
#23652=ORIENTED_EDGE('',*,*,#17111,.T.) ;
#23653=ORIENTED_EDGE('',*,*,#17112,.T.) ;
#23654=ORIENTED_EDGE('',*,*,#17097,.T.) ;
#23655=ORIENTED_EDGE('',*,*,#17113,.T.) ;
#23656=ORIENTED_EDGE('',*,*,#17114,.T.) ;
#23657=ORIENTED_EDGE('',*,*,#17115,.T.) ;
#23658=ORIENTED_EDGE('',*,*,#17093,.T.) ;
#23659=ORIENTED_EDGE('',*,*,#17116,.T.) ;
#23660=ORIENTED_EDGE('',*,*,#17117,.T.) ;
#23661=ORIENTED_EDGE('',*,*,#17118,.T.) ;
#23662=ORIENTED_EDGE('',*,*,#17089,.T.) ;
#23663=ORIENTED_EDGE('',*,*,#17119,.T.) ;
#23664=ORIENTED_EDGE('',*,*,#17120,.T.) ;
#23665=ORIENTED_EDGE('',*,*,#17121,.T.) ;
#23666=ORIENTED_EDGE('',*,*,#17085,.T.) ;
#23667=ORIENTED_EDGE('',*,*,#17122,.T.) ;
#23668=ORIENTED_EDGE('',*,*,#17123,.T.) ;
#23669=ORIENTED_EDGE('',*,*,#17124,.T.) ;
#23670=ORIENTED_EDGE('',*,*,#17081,.T.) ;
#23671=ORIENTED_EDGE('',*,*,#17125,.T.) ;
#23672=ORIENTED_EDGE('',*,*,#17126,.T.) ;
#23673=ORIENTED_EDGE('',*,*,#17127,.T.) ;
#23674=ORIENTED_EDGE('',*,*,#17077,.T.) ;
#23675=ORIENTED_EDGE('',*,*,#17128,.T.) ;
#23676=ORIENTED_EDGE('',*,*,#17129,.T.) ;
#23677=ORIENTED_EDGE('',*,*,#17130,.T.) ;
#23678=ORIENTED_EDGE('',*,*,#17073,.T.) ;
#23679=ORIENTED_EDGE('',*,*,#17131,.T.) ;
#23680=ORIENTED_EDGE('',*,*,#17132,.T.) ;
#23681=ORIENTED_EDGE('',*,*,#17133,.T.) ;
#23682=ORIENTED_EDGE('',*,*,#17069,.T.) ;
#23683=ORIENTED_EDGE('',*,*,#17109,.T.) ;
#23684=ORIENTED_EDGE('',*,*,#17102,.T.) ;
#23685=ORIENTED_EDGE('',*,*,#17106,.T.) ;
#23686=ORIENTED_EDGE('',*,*,#17065,.T.) ;
#23687=ORIENTED_EDGE('',*,*,#17060,.T.) ;
#23688=ORIENTED_EDGE('',*,*,#17061,.T.) ;
#23689=ORIENTED_EDGE('',*,*,#17071,.F.) ;
#23690=ORIENTED_EDGE('',*,*,#17134,.F.) ;
#23691=ORIENTED_EDGE('',*,*,#17135,.F.) ;
#23692=ORIENTED_EDGE('',*,*,#17136,.F.) ;
#23693=ORIENTED_EDGE('',*,*,#17072,.F.) ;
#23694=ORIENTED_EDGE('',*,*,#17136,.T.) ;
#23695=ORIENTED_EDGE('',*,*,#17137,.F.) ;
#23696=ORIENTED_EDGE('',*,*,#17131,.F.) ;
#23697=ORIENTED_EDGE('',*,*,#17132,.F.) ;
#23698=ORIENTED_EDGE('',*,*,#17137,.T.) ;
#23699=ORIENTED_EDGE('',*,*,#17135,.T.) ;
#23700=ORIENTED_EDGE('',*,*,#17138,.F.) ;
#23701=ORIENTED_EDGE('',*,*,#17070,.F.) ;
#23702=ORIENTED_EDGE('',*,*,#17133,.F.) ;
#23703=ORIENTED_EDGE('',*,*,#17138,.T.) ;
#23704=ORIENTED_EDGE('',*,*,#17134,.T.) ;
#23705=ORIENTED_EDGE('',*,*,#17129,.F.) ;
#23706=ORIENTED_EDGE('',*,*,#17139,.T.) ;
#23707=ORIENTED_EDGE('',*,*,#17140,.T.) ;
#23708=ORIENTED_EDGE('',*,*,#17141,.F.) ;
#23709=ORIENTED_EDGE('',*,*,#17130,.F.) ;
#23710=ORIENTED_EDGE('',*,*,#17141,.T.) ;
#23711=ORIENTED_EDGE('',*,*,#17142,.T.) ;
#23712=ORIENTED_EDGE('',*,*,#17074,.F.) ;
#23713=ORIENTED_EDGE('',*,*,#17075,.F.) ;
#23714=ORIENTED_EDGE('',*,*,#17142,.F.) ;
#23715=ORIENTED_EDGE('',*,*,#17140,.F.) ;
#23716=ORIENTED_EDGE('',*,*,#17143,.F.) ;
#23717=ORIENTED_EDGE('',*,*,#17128,.F.) ;
#23718=ORIENTED_EDGE('',*,*,#17076,.F.) ;
#23719=ORIENTED_EDGE('',*,*,#17143,.T.) ;
#23720=ORIENTED_EDGE('',*,*,#17139,.F.) ;
#23721=ORIENTED_EDGE('',*,*,#17079,.F.) ;
#23722=ORIENTED_EDGE('',*,*,#17144,.F.) ;
#23723=ORIENTED_EDGE('',*,*,#17145,.F.) ;
#23724=ORIENTED_EDGE('',*,*,#17146,.F.) ;
#23725=ORIENTED_EDGE('',*,*,#17080,.F.) ;
#23726=ORIENTED_EDGE('',*,*,#17146,.T.) ;
#23727=ORIENTED_EDGE('',*,*,#17147,.F.) ;
#23728=ORIENTED_EDGE('',*,*,#17125,.F.) ;
#23729=ORIENTED_EDGE('',*,*,#17126,.F.) ;
#23730=ORIENTED_EDGE('',*,*,#17147,.T.) ;
#23731=ORIENTED_EDGE('',*,*,#17145,.T.) ;
#23732=ORIENTED_EDGE('',*,*,#17148,.F.) ;
#23733=ORIENTED_EDGE('',*,*,#17078,.F.) ;
#23734=ORIENTED_EDGE('',*,*,#17127,.F.) ;
#23735=ORIENTED_EDGE('',*,*,#17148,.T.) ;
#23736=ORIENTED_EDGE('',*,*,#17144,.T.) ;
#23737=ORIENTED_EDGE('',*,*,#17123,.F.) ;
#23738=ORIENTED_EDGE('',*,*,#17149,.T.) ;
#23739=ORIENTED_EDGE('',*,*,#17150,.T.) ;
#23740=ORIENTED_EDGE('',*,*,#17151,.F.) ;
#23741=ORIENTED_EDGE('',*,*,#17124,.F.) ;
#23742=ORIENTED_EDGE('',*,*,#17151,.T.) ;
#23743=ORIENTED_EDGE('',*,*,#17152,.T.) ;
#23744=ORIENTED_EDGE('',*,*,#17082,.F.) ;
#23745=ORIENTED_EDGE('',*,*,#17083,.F.) ;
#23746=ORIENTED_EDGE('',*,*,#17152,.F.) ;
#23747=ORIENTED_EDGE('',*,*,#17150,.F.) ;
#23748=ORIENTED_EDGE('',*,*,#17153,.F.) ;
#23749=ORIENTED_EDGE('',*,*,#17122,.F.) ;
#23750=ORIENTED_EDGE('',*,*,#17084,.F.) ;
#23751=ORIENTED_EDGE('',*,*,#17153,.T.) ;
#23752=ORIENTED_EDGE('',*,*,#17149,.F.) ;
#23753=ORIENTED_EDGE('',*,*,#17087,.F.) ;
#23754=ORIENTED_EDGE('',*,*,#17154,.F.) ;
#23755=ORIENTED_EDGE('',*,*,#17155,.F.) ;
#23756=ORIENTED_EDGE('',*,*,#17156,.F.) ;
#23757=ORIENTED_EDGE('',*,*,#17088,.F.) ;
#23758=ORIENTED_EDGE('',*,*,#17156,.T.) ;
#23759=ORIENTED_EDGE('',*,*,#17157,.F.) ;
#23760=ORIENTED_EDGE('',*,*,#17119,.F.) ;
#23761=ORIENTED_EDGE('',*,*,#17120,.F.) ;
#23762=ORIENTED_EDGE('',*,*,#17157,.T.) ;
#23763=ORIENTED_EDGE('',*,*,#17155,.T.) ;
#23764=ORIENTED_EDGE('',*,*,#17158,.F.) ;
#23765=ORIENTED_EDGE('',*,*,#17086,.F.) ;
#23766=ORIENTED_EDGE('',*,*,#17121,.F.) ;
#23767=ORIENTED_EDGE('',*,*,#17158,.T.) ;
#23768=ORIENTED_EDGE('',*,*,#17154,.T.) ;
#23769=ORIENTED_EDGE('',*,*,#17117,.F.) ;
#23770=ORIENTED_EDGE('',*,*,#17159,.T.) ;
#23771=ORIENTED_EDGE('',*,*,#17160,.T.) ;
#23772=ORIENTED_EDGE('',*,*,#17161,.F.) ;
#23773=ORIENTED_EDGE('',*,*,#17118,.F.) ;
#23774=ORIENTED_EDGE('',*,*,#17161,.T.) ;
#23775=ORIENTED_EDGE('',*,*,#17162,.T.) ;
#23776=ORIENTED_EDGE('',*,*,#17090,.F.) ;
#23777=ORIENTED_EDGE('',*,*,#17091,.F.) ;
#23778=ORIENTED_EDGE('',*,*,#17162,.F.) ;
#23779=ORIENTED_EDGE('',*,*,#17160,.F.) ;
#23780=ORIENTED_EDGE('',*,*,#17163,.F.) ;
#23781=ORIENTED_EDGE('',*,*,#17116,.F.) ;
#23782=ORIENTED_EDGE('',*,*,#17092,.F.) ;
#23783=ORIENTED_EDGE('',*,*,#17163,.T.) ;
#23784=ORIENTED_EDGE('',*,*,#17159,.F.) ;
#23785=ORIENTED_EDGE('',*,*,#17095,.F.) ;
#23786=ORIENTED_EDGE('',*,*,#17164,.F.) ;
#23787=ORIENTED_EDGE('',*,*,#17165,.F.) ;
#23788=ORIENTED_EDGE('',*,*,#17166,.F.) ;
#23789=ORIENTED_EDGE('',*,*,#17096,.F.) ;
#23790=ORIENTED_EDGE('',*,*,#17166,.T.) ;
#23791=ORIENTED_EDGE('',*,*,#17167,.F.) ;
#23792=ORIENTED_EDGE('',*,*,#17113,.F.) ;
#23793=ORIENTED_EDGE('',*,*,#17114,.F.) ;
#23794=ORIENTED_EDGE('',*,*,#17167,.T.) ;
#23795=ORIENTED_EDGE('',*,*,#17165,.T.) ;
#23796=ORIENTED_EDGE('',*,*,#17168,.F.) ;
#23797=ORIENTED_EDGE('',*,*,#17094,.F.) ;
#23798=ORIENTED_EDGE('',*,*,#17115,.F.) ;
#23799=ORIENTED_EDGE('',*,*,#17168,.T.) ;
#23800=ORIENTED_EDGE('',*,*,#17164,.T.) ;
#23801=ORIENTED_EDGE('',*,*,#17169,.T.) ;
#23802=ORIENTED_EDGE('',*,*,#17099,.T.) ;
#23803=ORIENTED_EDGE('',*,*,#17170,.T.) ;
#23804=ORIENTED_EDGE('',*,*,#17171,.T.) ;
#23805=ORIENTED_EDGE('',*,*,#17172,.T.) ;
#23806=ORIENTED_EDGE('',*,*,#17170,.F.) ;
#23807=ORIENTED_EDGE('',*,*,#17098,.F.) ;
#23808=ORIENTED_EDGE('',*,*,#17112,.F.) ;
#23809=ORIENTED_EDGE('',*,*,#17173,.T.) ;
#23810=ORIENTED_EDGE('',*,*,#17171,.F.) ;
#23811=ORIENTED_EDGE('',*,*,#17172,.F.) ;
#23812=ORIENTED_EDGE('',*,*,#17111,.F.) ;
#23813=ORIENTED_EDGE('',*,*,#17100,.T.) ;
#23814=ORIENTED_EDGE('',*,*,#17169,.F.) ;
#23815=ORIENTED_EDGE('',*,*,#17173,.F.) ;
#23816=ORIENTED_EDGE('',*,*,#17110,.F.) ;
#28045=ADVANCED_FACE('',(#3310),#2152,.T.) ;
#28046=ADVANCED_FACE('',(#3311),#2153,.T.) ;
#28047=ADVANCED_FACE('',(#3312),#2154,.T.) ;
#28048=ADVANCED_FACE('',(#3313),#2155,.T.) ;
#28049=ADVANCED_FACE('',(#3314),#2156,.F.) ;
#28050=ADVANCED_FACE('',(#3315),#2157,.T.) ;
#28051=ADVANCED_FACE('',(#3316),#2158,.T.) ;
#28052=ADVANCED_FACE('',(#3317),#2159,.T.) ;
#28053=ADVANCED_FACE('',(#3318),#2160,.T.) ;
#28054=ADVANCED_FACE('',(#3319),#2161,.T.) ;
#28055=ADVANCED_FACE('',(#3320),#2162,.T.) ;
#28056=ADVANCED_FACE('',(#3321),#2163,.T.) ;
#28057=ADVANCED_FACE('',(#3322),#2164,.T.) ;
#28058=ADVANCED_FACE('',(#3323),#2165,.T.) ;
#28059=ADVANCED_FACE('',(#3324),#2166,.T.) ;
#28060=ADVANCED_FACE('',(#3325),#2167,.T.) ;
#28061=ADVANCED_FACE('',(#3326),#2168,.T.) ;
#28062=ADVANCED_FACE('',(#3327),#2169,.T.) ;
#28063=ADVANCED_FACE('',(#3328),#2170,.T.) ;
#28064=ADVANCED_FACE('',(#3329),#2171,.T.) ;
#28065=ADVANCED_FACE('',(#3330),#2172,.T.) ;
#28066=ADVANCED_FACE('',(#3331),#2173,.T.) ;
#28067=ADVANCED_FACE('',(#3332),#2174,.T.) ;
#28068=ADVANCED_FACE('',(#3333),#2175,.T.) ;
#28069=ADVANCED_FACE('',(#3334),#2176,.T.) ;
#28070=ADVANCED_FACE('',(#3335),#2177,.T.) ;
#28071=ADVANCED_FACE('',(#3336),#2178,.T.) ;
#28072=ADVANCED_FACE('',(#3337),#2179,.T.) ;
#28073=ADVANCED_FACE('',(#3338),#2180,.T.) ;
#28074=ADVANCED_FACE('',(#3339),#2181,.T.) ;
#28075=ADVANCED_FACE('',(#3340),#2182,.T.) ;
#28076=ADVANCED_FACE('',(#3341),#2183,.T.) ;
#28077=ADVANCED_FACE('',(#3342),#2184,.T.) ;
#28078=ADVANCED_FACE('',(#3343),#2185,.T.) ;
#28079=ADVANCED_FACE('',(#3344),#2186,.T.) ;
#28080=ADVANCED_FACE('',(#3345),#2187,.T.) ;
#28081=ADVANCED_FACE('',(#3346),#2188,.T.) ;
#28082=ADVANCED_FACE('',(#3347),#2189,.T.) ;
#28083=ADVANCED_FACE('',(#3348),#2190,.F.) ;
#28084=ADVANCED_FACE('',(#3349),#2191,.F.) ;
#28085=ADVANCED_FACE('',(#3350),#2192,.F.) ;
#28086=ADVANCED_FACE('',(#3351),#2193,.F.) ;
#28671=CLOSED_SHELL('',(#28045,#28046,#28047,#28048,#28049,#28050,#28051,
#28052,#28053,#28054,#28055,#28056,#28057,#28058,#28059,#28060,#28061,#28062,
#28063,#28064,#28065,#28066,#28067,#28068,#28069,#28070,#28071,#28072,#28073,
#28074,#28075,#28076,#28077,#28078,#28079,#28080,#28081,#28082,#28083,#28084,
#28085,#28086)) ;
#30765=AXIS2_PLACEMENT_3D('',#46557,#37434,#37435) ;
#30766=AXIS2_PLACEMENT_3D('',#46558,#37436,#37437) ;
#30767=AXIS2_PLACEMENT_3D('',#46567,#37442,#37443) ;
#30768=AXIS2_PLACEMENT_3D('',#46573,#37447,#37448) ;
#30769=AXIS2_PLACEMENT_3D('',#46577,#37451,#37452) ;
#30770=AXIS2_PLACEMENT_3D('',#46581,#37455,#37456) ;
#30771=AXIS2_PLACEMENT_3D('',#46655,#37494,#37495) ;
#30772=AXIS2_PLACEMENT_3D('',#46664,#37500,#37501) ;
#30773=AXIS2_PLACEMENT_3D('',#46667,#37504,#37505) ;
#30774=AXIS2_PLACEMENT_3D('',#46669,#37507,#37508) ;
#30775=AXIS2_PLACEMENT_3D('',#46671,#37510,#37511) ;
#30776=AXIS2_PLACEMENT_3D('',#46712,#37536,#37537) ;
#30777=AXIS2_PLACEMENT_3D('',#46718,#37541,#37542) ;
#30778=AXIS2_PLACEMENT_3D('',#46720,#37544,#37545) ;
#30779=AXIS2_PLACEMENT_3D('',#46722,#37547,#37548) ;
#30780=AXIS2_PLACEMENT_3D('',#46723,#37549,#37550) ;
#30781=AXIS2_PLACEMENT_3D('',#46729,#37554,#37555) ;
#30782=AXIS2_PLACEMENT_3D('',#46731,#37557,#37558) ;
#30783=AXIS2_PLACEMENT_3D('',#46733,#37560,#37561) ;
#30784=AXIS2_PLACEMENT_3D('',#46734,#37562,#37563) ;
#30785=AXIS2_PLACEMENT_3D('',#46740,#37567,#37568) ;
#30786=AXIS2_PLACEMENT_3D('',#46742,#37570,#37571) ;
#30787=AXIS2_PLACEMENT_3D('',#46744,#37573,#37574) ;
#30788=AXIS2_PLACEMENT_3D('',#46745,#37575,#37576) ;
#30789=AXIS2_PLACEMENT_3D('',#46751,#37580,#37581) ;
#30790=AXIS2_PLACEMENT_3D('',#46753,#37583,#37584) ;
#30791=AXIS2_PLACEMENT_3D('',#46755,#37586,#37587) ;
#30792=AXIS2_PLACEMENT_3D('',#46756,#37588,#37589) ;
#30793=AXIS2_PLACEMENT_3D('',#46762,#37593,#37594) ;
#30794=AXIS2_PLACEMENT_3D('',#46764,#37596,#37597) ;
#30795=AXIS2_PLACEMENT_3D('',#46766,#37599,#37600) ;
#30796=AXIS2_PLACEMENT_3D('',#46767,#37601,#37602) ;
#30797=AXIS2_PLACEMENT_3D('',#46773,#37606,#37607) ;
#30798=AXIS2_PLACEMENT_3D('',#46775,#37609,#37610) ;
#30799=AXIS2_PLACEMENT_3D('',#46777,#37612,#37613) ;
#30800=AXIS2_PLACEMENT_3D('',#46778,#37614,#37615) ;
#30801=AXIS2_PLACEMENT_3D('',#46784,#37619,#37620) ;
#30802=AXIS2_PLACEMENT_3D('',#46786,#37622,#37623) ;
#30803=AXIS2_PLACEMENT_3D('',#46788,#37625,#37626) ;
#30804=AXIS2_PLACEMENT_3D('',#46789,#37627,#37628) ;
#30805=AXIS2_PLACEMENT_3D('',#46795,#37632,#37633) ;
#30806=AXIS2_PLACEMENT_3D('',#46797,#37635,#37636) ;
#30807=AXIS2_PLACEMENT_3D('',#46799,#37638,#37639) ;
#37434=DIRECTION('axis',(0.,0.,1.)) ;
#37435=DIRECTION('refdir',(1.,0.,0.)) ;
#37436=DIRECTION('center_axis',(0.,0.,1.)) ;
#37437=DIRECTION('ref_axis',(1.,0.,0.)) ;
#37438=DIRECTION('',(-1.,0.,0.)) ;
#37439=DIRECTION('',(0.,-1.,0.)) ;
#37440=DIRECTION('',(1.,0.,0.)) ;
#37441=DIRECTION('',(0.,1.,0.)) ;
#37442=DIRECTION('center_axis',(1.,0.,0.)) ;
#37443=DIRECTION('ref_axis',(0.,0.,-1.)) ;
#37444=DIRECTION('',(0.,0.,1.)) ;
#37445=DIRECTION('',(0.,0.,-1.)) ;
#37446=DIRECTION('',(0.,1.,0.)) ;
#37447=DIRECTION('center_axis',(0.,-1.,0.)) ;
#37448=DIRECTION('ref_axis',(0.,0.,-1.)) ;
#37449=DIRECTION('',(1.,0.,0.)) ;
#37450=DIRECTION('',(0.,0.,-1.)) ;
#37451=DIRECTION('center_axis',(-1.,0.,0.)) ;
#37452=DIRECTION('ref_axis',(0.,0.,1.)) ;
#37453=DIRECTION('',(0.,0.,-1.)) ;
#37454=DIRECTION('',(0.,-1.,0.)) ;
#37455=DIRECTION('center_axis',(0.,1.,0.)) ;
#37456=DIRECTION('ref_axis',(0.,0.,1.)) ;
#37457=DIRECTION('',(1.,0.,0.)) ;
#37458=DIRECTION('',(0.,0.,-1.)) ;
#37459=DIRECTION('',(-1.,0.,0.)) ;
#37460=DIRECTION('',(0.,0.,1.)) ;
#37461=DIRECTION('',(1.,0.,0.)) ;
#37462=DIRECTION('',(0.,0.,-1.)) ;
#37463=DIRECTION('',(-1.,0.,0.)) ;
#37464=DIRECTION('',(0.,0.,1.)) ;
#37465=DIRECTION('',(1.,0.,0.)) ;
#37466=DIRECTION('',(0.,0.,-1.)) ;
#37467=DIRECTION('',(-1.,0.,0.)) ;
#37468=DIRECTION('',(0.,0.,1.)) ;
#37469=DIRECTION('',(1.,0.,0.)) ;
#37470=DIRECTION('',(0.,0.,-1.)) ;
#37471=DIRECTION('',(-1.,0.,0.)) ;
#37472=DIRECTION('',(0.,0.,1.)) ;
#37473=DIRECTION('',(1.,0.,0.)) ;
#37474=DIRECTION('',(0.,0.,-1.)) ;
#37475=DIRECTION('',(-1.,0.,0.)) ;
#37476=DIRECTION('',(0.,0.,1.)) ;
#37477=DIRECTION('',(1.,0.,0.)) ;
#37478=DIRECTION('',(0.,0.,-1.)) ;
#37479=DIRECTION('',(-1.,0.,0.)) ;
#37480=DIRECTION('',(0.,0.,1.)) ;
#37481=DIRECTION('',(1.,0.,0.)) ;
#37482=DIRECTION('',(0.,0.,-1.)) ;
#37483=DIRECTION('',(-1.,0.,0.)) ;
#37484=DIRECTION('',(0.,0.,1.)) ;
#37485=DIRECTION('',(1.,0.,0.)) ;
#37486=DIRECTION('',(0.,0.,-1.)) ;
#37487=DIRECTION('',(-1.,0.,0.)) ;
#37488=DIRECTION('',(0.,0.,1.)) ;
#37489=DIRECTION('',(1.,0.,0.)) ;
#37490=DIRECTION('',(0.,0.,-1.)) ;
#37491=DIRECTION('',(-1.,0.,0.)) ;
#37492=DIRECTION('',(0.,0.,-1.)) ;
#37493=DIRECTION('',(1.,0.,0.)) ;
#37494=DIRECTION('center_axis',(0.,-1.,0.)) ;
#37495=DIRECTION('ref_axis',(0.,0.,-1.)) ;
#37496=DIRECTION('',(1.,0.,0.)) ;
#37497=DIRECTION('',(0.,0.,-1.)) ;
#37498=DIRECTION('',(1.,0.,0.)) ;
#37499=DIRECTION('',(0.,0.,-1.)) ;
#37500=DIRECTION('center_axis',(-1.,0.,0.)) ;
#37501=DIRECTION('ref_axis',(0.,0.,1.)) ;
#37502=DIRECTION('',(0.,-1.,0.)) ;
#37503=DIRECTION('',(0.,-1.,0.)) ;
#37504=DIRECTION('center_axis',(0.,0.,1.)) ;
#37505=DIRECTION('ref_axis',(1.,0.,0.)) ;
#37506=DIRECTION('',(0.,1.,0.)) ;
#37507=DIRECTION('center_axis',(1.,0.,0.)) ;
#37508=DIRECTION('ref_axis',(0.,0.,-1.)) ;
#37509=DIRECTION('',(0.,1.,0.)) ;
#37510=DIRECTION('center_axis',(0.,0.,1.)) ;
#37511=DIRECTION('ref_axis',(1.,0.,0.)) ;
#37512=DIRECTION('',(0.,1.,0.)) ;
#37513=DIRECTION('',(-1.,0.,0.)) ;
#37514=DIRECTION('',(0.,-1.,0.)) ;
#37515=DIRECTION('',(0.,1.,0.)) ;
#37516=DIRECTION('',(1.,0.,0.)) ;
#37517=DIRECTION('',(0.,-1.,0.)) ;
#37518=DIRECTION('',(0.,1.,0.)) ;
#37519=DIRECTION('',(1.,0.,0.)) ;
#37520=DIRECTION('',(0.,-1.,0.)) ;
#37521=DIRECTION('',(0.,1.,0.)) ;
#37522=DIRECTION('',(1.,0.,0.)) ;
#37523=DIRECTION('',(0.,-1.,0.)) ;
#37524=DIRECTION('',(0.,1.,0.)) ;
#37525=DIRECTION('',(1.,0.,0.)) ;
#37526=DIRECTION('',(0.,-1.,0.)) ;
#37527=DIRECTION('',(0.,1.,0.)) ;
#37528=DIRECTION('',(1.,0.,0.)) ;
#37529=DIRECTION('',(0.,-1.,0.)) ;
#37530=DIRECTION('',(0.,1.,0.)) ;
#37531=DIRECTION('',(1.,0.,0.)) ;
#37532=DIRECTION('',(0.,-1.,0.)) ;
#37533=DIRECTION('',(0.,1.,0.)) ;
#37534=DIRECTION('',(1.,0.,0.)) ;
#37535=DIRECTION('',(0.,-1.,0.)) ;
#37536=DIRECTION('center_axis',(0.,0.,1.)) ;
#37537=DIRECTION('ref_axis',(1.,0.,0.)) ;
#37538=DIRECTION('',(0.,-1.,0.)) ;
#37539=DIRECTION('',(1.,0.,0.)) ;
#37540=DIRECTION('',(0.,1.,0.)) ;
#37541=DIRECTION('center_axis',(1.,0.,0.)) ;
#37542=DIRECTION('ref_axis',(0.,0.,-1.)) ;
#37543=DIRECTION('',(0.,0.,-1.)) ;
#37544=DIRECTION('center_axis',(0.,-1.,0.)) ;
#37545=DIRECTION('ref_axis',(0.,0.,-1.)) ;
#37546=DIRECTION('',(0.,0.,-1.)) ;
#37547=DIRECTION('center_axis',(-1.,0.,0.)) ;
#37548=DIRECTION('ref_axis',(0.,0.,1.)) ;
#37549=DIRECTION('center_axis',(0.,-1.,0.)) ;
#37550=DIRECTION('ref_axis',(0.,0.,-1.)) ;
#37551=DIRECTION('',(0.,0.,-1.)) ;
#37552=DIRECTION('',(1.,0.,0.)) ;
#37553=DIRECTION('',(0.,0.,-1.)) ;
#37554=DIRECTION('center_axis',(-1.,0.,0.)) ;
#37555=DIRECTION('ref_axis',(0.,0.,1.)) ;
#37556=DIRECTION('',(0.,-1.,0.)) ;
#37557=DIRECTION('center_axis',(0.,0.,1.)) ;
#37558=DIRECTION('ref_axis',(1.,0.,0.)) ;
#37559=DIRECTION('',(0.,1.,0.)) ;
#37560=DIRECTION('center_axis',(1.,0.,0.)) ;
#37561=DIRECTION('ref_axis',(0.,0.,-1.)) ;
#37562=DIRECTION('center_axis',(0.,0.,1.)) ;
#37563=DIRECTION('ref_axis',(1.,0.,0.)) ;
#37564=DIRECTION('',(0.,-1.,0.)) ;
#37565=DIRECTION('',(1.,0.,0.)) ;
#37566=DIRECTION('',(0.,1.,0.)) ;
#37567=DIRECTION('center_axis',(1.,0.,0.)) ;
#37568=DIRECTION('ref_axis',(0.,0.,-1.)) ;
#37569=DIRECTION('',(0.,0.,-1.)) ;
#37570=DIRECTION('center_axis',(0.,-1.,0.)) ;
#37571=DIRECTION('ref_axis',(0.,0.,-1.)) ;
#37572=DIRECTION('',(0.,0.,-1.)) ;
#37573=DIRECTION('center_axis',(-1.,0.,0.)) ;
#37574=DIRECTION('ref_axis',(0.,0.,1.)) ;
#37575=DIRECTION('center_axis',(0.,-1.,0.)) ;
#37576=DIRECTION('ref_axis',(0.,0.,-1.)) ;
#37577=DIRECTION('',(0.,0.,-1.)) ;
#37578=DIRECTION('',(1.,0.,0.)) ;
#37579=DIRECTION('',(0.,0.,-1.)) ;
#37580=DIRECTION('center_axis',(-1.,0.,0.)) ;
#37581=DIRECTION('ref_axis',(0.,0.,1.)) ;
#37582=DIRECTION('',(0.,-1.,0.)) ;
#37583=DIRECTION('center_axis',(0.,0.,1.)) ;
#37584=DIRECTION('ref_axis',(1.,0.,0.)) ;
#37585=DIRECTION('',(0.,1.,0.)) ;
#37586=DIRECTION('center_axis',(1.,0.,0.)) ;
#37587=DIRECTION('ref_axis',(0.,0.,-1.)) ;
#37588=DIRECTION('center_axis',(0.,0.,1.)) ;
#37589=DIRECTION('ref_axis',(1.,0.,0.)) ;
#37590=DIRECTION('',(0.,-1.,0.)) ;
#37591=DIRECTION('',(1.,0.,0.)) ;
#37592=DIRECTION('',(0.,1.,0.)) ;
#37593=DIRECTION('center_axis',(1.,0.,0.)) ;
#37594=DIRECTION('ref_axis',(0.,0.,-1.)) ;
#37595=DIRECTION('',(0.,0.,-1.)) ;
#37596=DIRECTION('center_axis',(0.,-1.,0.)) ;
#37597=DIRECTION('ref_axis',(0.,0.,-1.)) ;
#37598=DIRECTION('',(0.,0.,-1.)) ;
#37599=DIRECTION('center_axis',(-1.,0.,0.)) ;
#37600=DIRECTION('ref_axis',(0.,0.,1.)) ;
#37601=DIRECTION('center_axis',(0.,-1.,0.)) ;
#37602=DIRECTION('ref_axis',(0.,0.,-1.)) ;
#37603=DIRECTION('',(0.,0.,-1.)) ;
#37604=DIRECTION('',(1.,0.,0.)) ;
#37605=DIRECTION('',(0.,0.,-1.)) ;
#37606=DIRECTION('center_axis',(-1.,0.,0.)) ;
#37607=DIRECTION('ref_axis',(0.,0.,1.)) ;
#37608=DIRECTION('',(0.,-1.,0.)) ;
#37609=DIRECTION('center_axis',(0.,0.,1.)) ;
#37610=DIRECTION('ref_axis',(1.,0.,0.)) ;
#37611=DIRECTION('',(0.,1.,0.)) ;
#37612=DIRECTION('center_axis',(1.,0.,0.)) ;
#37613=DIRECTION('ref_axis',(0.,0.,-1.)) ;
#37614=DIRECTION('center_axis',(0.,0.,1.)) ;
#37615=DIRECTION('ref_axis',(1.,0.,0.)) ;
#37616=DIRECTION('',(0.,-1.,0.)) ;
#37617=DIRECTION('',(1.,0.,0.)) ;
#37618=DIRECTION('',(0.,1.,0.)) ;
#37619=DIRECTION('center_axis',(1.,0.,0.)) ;
#37620=DIRECTION('ref_axis',(0.,0.,-1.)) ;
#37621=DIRECTION('',(0.,0.,-1.)) ;
#37622=DIRECTION('center_axis',(0.,-1.,0.)) ;
#37623=DIRECTION('ref_axis',(0.,0.,-1.)) ;
#37624=DIRECTION('',(0.,0.,-1.)) ;
#37625=DIRECTION('center_axis',(-1.,0.,0.)) ;
#37626=DIRECTION('ref_axis',(0.,0.,1.)) ;
#37627=DIRECTION('center_axis',(0.,0.,1.)) ;
#37628=DIRECTION('ref_axis',(1.,0.,0.)) ;
#37629=DIRECTION('',(0.,-1.,0.)) ;
#37630=DIRECTION('',(0.,1.,0.)) ;
#37631=DIRECTION('',(1.,0.,0.)) ;
#37632=DIRECTION('center_axis',(1.,0.,0.)) ;
#37633=DIRECTION('ref_axis',(0.,0.,-1.)) ;
#37634=DIRECTION('',(0.,0.,-1.)) ;
#37635=DIRECTION('center_axis',(0.,-1.,0.)) ;
#37636=DIRECTION('ref_axis',(0.,0.,-1.)) ;
#37637=DIRECTION('',(0.,0.,-1.)) ;
#37638=DIRECTION('center_axis',(-1.,0.,0.)) ;
#37639=DIRECTION('ref_axis',(0.,0.,1.)) ;
#46557=CARTESIAN_POINT('',(0.,0.,0.)) ;
#46558=CARTESIAN_POINT('Origin',(24.2,6.35,42.5)) ;
#46559=CARTESIAN_POINT('',(24.3,6.,42.5)) ;
#46560=CARTESIAN_POINT('',(24.1,6.,42.5)) ;
#46561=CARTESIAN_POINT('',(22.35,6.,42.5)) ;
#46562=CARTESIAN_POINT('',(24.3,6.8,42.5)) ;
#46563=CARTESIAN_POINT('',(24.3,6.35,42.5)) ;
#46564=CARTESIAN_POINT('',(24.1,6.8,42.5)) ;
#46565=CARTESIAN_POINT('',(24.2,6.8,42.5)) ;
#46566=CARTESIAN_POINT('',(24.1,6.35,42.5)) ;
#46567=CARTESIAN_POINT('Origin',(24.1,6.35,42.6)) ;
#46568=CARTESIAN_POINT('',(24.1,6.,42.6)) ;
#46569=CARTESIAN_POINT('',(24.1,6.,42.55)) ;
#46570=CARTESIAN_POINT('',(24.1,6.8,42.6)) ;
#46571=CARTESIAN_POINT('',(24.1,6.8,42.6)) ;
#46572=CARTESIAN_POINT('',(24.1,6.475,42.6)) ;
#46573=CARTESIAN_POINT('Origin',(24.2,6.8,42.6)) ;
#46574=CARTESIAN_POINT('',(24.3,6.8,42.6)) ;
#46575=CARTESIAN_POINT('',(22.35,6.8,42.6)) ;
#46576=CARTESIAN_POINT('',(24.3,6.8,42.6)) ;
#46577=CARTESIAN_POINT('Origin',(24.3,6.35,42.6)) ;
#46578=CARTESIAN_POINT('',(24.3,6.,42.6)) ;
#46579=CARTESIAN_POINT('',(24.3,6.,42.55)) ;
#46580=CARTESIAN_POINT('',(24.3,6.475,42.6)) ;
#46581=CARTESIAN_POINT('Origin',(20.5,6.,42.5)) ;
#46582=CARTESIAN_POINT('',(23.4,6.,42.6)) ;
#46583=CARTESIAN_POINT('',(20.5,6.,42.6)) ;
#46584=CARTESIAN_POINT('',(23.4,6.,42.5)) ;
#46585=CARTESIAN_POINT('',(23.4,6.,42.55)) ;
#46586=CARTESIAN_POINT('',(23.2,6.,42.5)) ;
#46587=CARTESIAN_POINT('',(21.9,6.,42.5)) ;
#46588=CARTESIAN_POINT('',(23.2,6.,42.6)) ;
#46589=CARTESIAN_POINT('',(23.2,6.,42.55)) ;
#46590=CARTESIAN_POINT('',(22.5,6.,42.6)) ;
#46591=CARTESIAN_POINT('',(20.5,6.,42.6)) ;
#46592=CARTESIAN_POINT('',(22.5,6.,42.5)) ;
#46593=CARTESIAN_POINT('',(22.5,6.,42.55)) ;
#46594=CARTESIAN_POINT('',(22.3,6.,42.5)) ;
#46595=CARTESIAN_POINT('',(21.45,6.,42.5)) ;
#46596=CARTESIAN_POINT('',(22.3,6.,42.6)) ;
#46597=CARTESIAN_POINT('',(22.3,6.,42.55)) ;
#46598=CARTESIAN_POINT('',(21.6,6.,42.6)) ;
#46599=CARTESIAN_POINT('',(20.5,6.,42.6)) ;
#46600=CARTESIAN_POINT('',(21.6,6.,42.5)) ;
#46601=CARTESIAN_POINT('',(21.6,6.,42.55)) ;
#46602=CARTESIAN_POINT('',(21.4,6.,42.5)) ;
#46603=CARTESIAN_POINT('',(21.,6.,42.5)) ;
#46604=CARTESIAN_POINT('',(21.4,6.,42.6)) ;
#46605=CARTESIAN_POINT('',(21.4,6.,42.55)) ;
#46606=CARTESIAN_POINT('',(20.7,6.,42.6)) ;
#46607=CARTESIAN_POINT('',(20.5,6.,42.6)) ;
#46608=CARTESIAN_POINT('',(20.7,6.,42.5)) ;
#46609=CARTESIAN_POINT('',(20.7,6.,42.55)) ;
#46610=CARTESIAN_POINT('',(20.5,6.,42.5)) ;
#46611=CARTESIAN_POINT('',(20.55,6.,42.5)) ;
#46612=CARTESIAN_POINT('',(20.5,6.,42.6)) ;
#46613=CARTESIAN_POINT('',(20.5,6.,42.55)) ;
#46614=CARTESIAN_POINT('',(19.8,6.,42.6)) ;
#46615=CARTESIAN_POINT('',(20.5,6.,42.6)) ;
#46616=CARTESIAN_POINT('',(19.8,6.,42.5)) ;
#46617=CARTESIAN_POINT('',(19.8,6.,42.55)) ;
#46618=CARTESIAN_POINT('',(19.6,6.,42.5)) ;
#46619=CARTESIAN_POINT('',(20.1,6.,42.5)) ;
#46620=CARTESIAN_POINT('',(19.6,6.,42.6)) ;
#46621=CARTESIAN_POINT('',(19.6,6.,42.55)) ;
#46622=CARTESIAN_POINT('',(18.9,6.,42.6)) ;
#46623=CARTESIAN_POINT('',(20.5,6.,42.6)) ;
#46624=CARTESIAN_POINT('',(18.9,6.,42.5)) ;
#46625=CARTESIAN_POINT('',(18.9,6.,42.55)) ;
#46626=CARTESIAN_POINT('',(18.7,6.,42.5)) ;
#46627=CARTESIAN_POINT('',(19.65,6.,42.5)) ;
#46628=CARTESIAN_POINT('',(18.7,6.,42.6)) ;
#46629=CARTESIAN_POINT('',(18.7,6.,42.55)) ;
#46630=CARTESIAN_POINT('',(18.,6.,42.6)) ;
#46631=CARTESIAN_POINT('',(20.5,6.,42.6)) ;
#46632=CARTESIAN_POINT('',(18.,6.,42.5)) ;
#46633=CARTESIAN_POINT('',(18.,6.,42.55)) ;
#46634=CARTESIAN_POINT('',(17.8,6.,42.5)) ;
#46635=CARTESIAN_POINT('',(19.2,6.,42.5)) ;
#46636=CARTESIAN_POINT('',(17.8,6.,42.6)) ;
#46637=CARTESIAN_POINT('',(17.8,6.,42.55)) ;
#46638=CARTESIAN_POINT('',(17.1,6.,42.6)) ;
#46639=CARTESIAN_POINT('',(20.5,6.,42.6)) ;
#46640=CARTESIAN_POINT('',(17.1,6.,42.5)) ;
#46641=CARTESIAN_POINT('',(17.1,6.,42.55)) ;
#46642=CARTESIAN_POINT('',(16.9,6.,42.5)) ;
#46643=CARTESIAN_POINT('',(18.75,6.,42.5)) ;
#46644=CARTESIAN_POINT('',(16.9,6.,42.6)) ;
#46645=CARTESIAN_POINT('',(16.9,6.,42.55)) ;
#46646=CARTESIAN_POINT('',(16.5,6.,42.6)) ;
#46647=CARTESIAN_POINT('',(20.5,6.,42.6)) ;
#46648=CARTESIAN_POINT('',(16.5,6.,42.4)) ;
#46649=CARTESIAN_POINT('',(16.5,6.,42.5)) ;
#46650=CARTESIAN_POINT('',(24.5,6.,42.4)) ;
#46651=CARTESIAN_POINT('',(20.5,6.,42.4)) ;
#46652=CARTESIAN_POINT('',(24.5,6.,42.6)) ;
#46653=CARTESIAN_POINT('',(24.5,6.,42.5)) ;
#46654=CARTESIAN_POINT('',(20.5,6.,42.6)) ;
#46655=CARTESIAN_POINT('Origin',(23.3,6.8,42.6)) ;
#46656=CARTESIAN_POINT('',(23.2,6.8,42.6)) ;
#46657=CARTESIAN_POINT('',(23.4,6.8,42.6)) ;
#46658=CARTESIAN_POINT('',(21.9,6.8,42.6)) ;
#46659=CARTESIAN_POINT('',(23.2,6.8,42.5)) ;
#46660=CARTESIAN_POINT('',(23.2,6.8,42.6)) ;
#46661=CARTESIAN_POINT('',(23.4,6.8,42.5)) ;
#46662=CARTESIAN_POINT('',(23.3,6.8,42.5)) ;
#46663=CARTESIAN_POINT('',(23.4,6.8,42.6)) ;
#46664=CARTESIAN_POINT('Origin',(23.4,6.35,42.6)) ;
#46665=CARTESIAN_POINT('',(23.4,6.475,42.6)) ;
#46666=CARTESIAN_POINT('',(23.4,6.35,42.5)) ;
#46667=CARTESIAN_POINT('Origin',(23.3,6.35,42.5)) ;
#46668=CARTESIAN_POINT('',(23.2,6.35,42.5)) ;
#46669=CARTESIAN_POINT('Origin',(23.2,6.35,42.6)) ;
#46670=CARTESIAN_POINT('',(23.2,6.475,42.6)) ;
#46671=CARTESIAN_POINT('Origin',(20.5,6.6,42.6)) ;
#46672=CARTESIAN_POINT('',(24.5,7.2,42.6)) ;
#46673=CARTESIAN_POINT('',(24.5,6.6,42.6)) ;
#46674=CARTESIAN_POINT('',(16.5,7.2,42.6)) ;
#46675=CARTESIAN_POINT('',(20.5,7.2,42.6)) ;
#46676=CARTESIAN_POINT('',(16.5,6.6,42.6)) ;
#46677=CARTESIAN_POINT('',(16.9,6.8,42.6)) ;
#46678=CARTESIAN_POINT('',(16.9,6.475,42.6)) ;
#46679=CARTESIAN_POINT('',(17.1,6.8,42.6)) ;
#46680=CARTESIAN_POINT('',(18.75,6.8,42.6)) ;
#46681=CARTESIAN_POINT('',(17.1,6.475,42.6)) ;
#46682=CARTESIAN_POINT('',(17.8,6.8,42.6)) ;
#46683=CARTESIAN_POINT('',(17.8,6.475,42.6)) ;
#46684=CARTESIAN_POINT('',(18.,6.8,42.6)) ;
#46685=CARTESIAN_POINT('',(19.2,6.8,42.6)) ;
#46686=CARTESIAN_POINT('',(18.,6.475,42.6)) ;
#46687=CARTESIAN_POINT('',(18.7,6.8,42.6)) ;
#46688=CARTESIAN_POINT('',(18.7,6.475,42.6)) ;
#46689=CARTESIAN_POINT('',(18.9,6.8,42.6)) ;
#46690=CARTESIAN_POINT('',(19.65,6.8,42.6)) ;
#46691=CARTESIAN_POINT('',(18.9,6.475,42.6)) ;
#46692=CARTESIAN_POINT('',(19.6,6.8,42.6)) ;
#46693=CARTESIAN_POINT('',(19.6,6.475,42.6)) ;
#46694=CARTESIAN_POINT('',(19.8,6.8,42.6)) ;
#46695=CARTESIAN_POINT('',(20.1,6.8,42.6)) ;
#46696=CARTESIAN_POINT('',(19.8,6.475,42.6)) ;
#46697=CARTESIAN_POINT('',(20.5,6.8,42.6)) ;
#46698=CARTESIAN_POINT('',(20.5,6.475,42.6)) ;
#46699=CARTESIAN_POINT('',(20.7,6.8,42.6)) ;
#46700=CARTESIAN_POINT('',(20.55,6.8,42.6)) ;
#46701=CARTESIAN_POINT('',(20.7,6.475,42.6)) ;
#46702=CARTESIAN_POINT('',(21.4,6.8,42.6)) ;
#46703=CARTESIAN_POINT('',(21.4,6.475,42.6)) ;
#46704=CARTESIAN_POINT('',(21.6,6.8,42.6)) ;
#46705=CARTESIAN_POINT('',(21.,6.8,42.6)) ;
#46706=CARTESIAN_POINT('',(21.6,6.475,42.6)) ;
#46707=CARTESIAN_POINT('',(22.3,6.8,42.6)) ;
#46708=CARTESIAN_POINT('',(22.3,6.475,42.6)) ;
#46709=CARTESIAN_POINT('',(22.5,6.8,42.6)) ;
#46710=CARTESIAN_POINT('',(21.45,6.8,42.6)) ;
#46711=CARTESIAN_POINT('',(22.5,6.475,42.6)) ;
#46712=CARTESIAN_POINT('Origin',(22.4,6.35,42.5)) ;
#46713=CARTESIAN_POINT('',(22.5,6.8,42.5)) ;
#46714=CARTESIAN_POINT('',(22.5,6.35,42.5)) ;
#46715=CARTESIAN_POINT('',(22.3,6.8,42.5)) ;
#46716=CARTESIAN_POINT('',(22.4,6.8,42.5)) ;
#46717=CARTESIAN_POINT('',(22.3,6.35,42.5)) ;
#46718=CARTESIAN_POINT('Origin',(22.3,6.35,42.6)) ;
#46719=CARTESIAN_POINT('',(22.3,6.8,42.6)) ;
#46720=CARTESIAN_POINT('Origin',(22.4,6.8,42.6)) ;
#46721=CARTESIAN_POINT('',(22.5,6.8,42.6)) ;
#46722=CARTESIAN_POINT('Origin',(22.5,6.35,42.6)) ;
#46723=CARTESIAN_POINT('Origin',(21.5,6.8,42.6)) ;
#46724=CARTESIAN_POINT('',(21.4,6.8,42.5)) ;
#46725=CARTESIAN_POINT('',(21.4,6.8,42.6)) ;
#46726=CARTESIAN_POINT('',(21.6,6.8,42.5)) ;
#46727=CARTESIAN_POINT('',(21.5,6.8,42.5)) ;
#46728=CARTESIAN_POINT('',(21.6,6.8,42.6)) ;
#46729=CARTESIAN_POINT('Origin',(21.6,6.35,42.6)) ;
#46730=CARTESIAN_POINT('',(21.6,6.35,42.5)) ;
#46731=CARTESIAN_POINT('Origin',(21.5,6.35,42.5)) ;
#46732=CARTESIAN_POINT('',(21.4,6.35,42.5)) ;
#46733=CARTESIAN_POINT('Origin',(21.4,6.35,42.6)) ;
#46734=CARTESIAN_POINT('Origin',(20.6,6.35,42.5)) ;
#46735=CARTESIAN_POINT('',(20.7,6.8,42.5)) ;
#46736=CARTESIAN_POINT('',(20.7,6.35,42.5)) ;
#46737=CARTESIAN_POINT('',(20.5,6.8,42.5)) ;
#46738=CARTESIAN_POINT('',(20.6,6.8,42.5)) ;
#46739=CARTESIAN_POINT('',(20.5,6.35,42.5)) ;
#46740=CARTESIAN_POINT('Origin',(20.5,6.35,42.6)) ;
#46741=CARTESIAN_POINT('',(20.5,6.8,42.6)) ;
#46742=CARTESIAN_POINT('Origin',(20.6,6.8,42.6)) ;
#46743=CARTESIAN_POINT('',(20.7,6.8,42.6)) ;
#46744=CARTESIAN_POINT('Origin',(20.7,6.35,42.6)) ;
#46745=CARTESIAN_POINT('Origin',(19.7,6.8,42.6)) ;
#46746=CARTESIAN_POINT('',(19.6,6.8,42.5)) ;
#46747=CARTESIAN_POINT('',(19.6,6.8,42.6)) ;
#46748=CARTESIAN_POINT('',(19.8,6.8,42.5)) ;
#46749=CARTESIAN_POINT('',(19.7,6.8,42.5)) ;
#46750=CARTESIAN_POINT('',(19.8,6.8,42.6)) ;
#46751=CARTESIAN_POINT('Origin',(19.8,6.35,42.6)) ;
#46752=CARTESIAN_POINT('',(19.8,6.35,42.5)) ;
#46753=CARTESIAN_POINT('Origin',(19.7,6.35,42.5)) ;
#46754=CARTESIAN_POINT('',(19.6,6.35,42.5)) ;
#46755=CARTESIAN_POINT('Origin',(19.6,6.35,42.6)) ;
#46756=CARTESIAN_POINT('Origin',(18.8,6.35,42.5)) ;
#46757=CARTESIAN_POINT('',(18.9,6.8,42.5)) ;
#46758=CARTESIAN_POINT('',(18.9,6.35,42.5)) ;
#46759=CARTESIAN_POINT('',(18.7,6.8,42.5)) ;
#46760=CARTESIAN_POINT('',(18.8,6.8,42.5)) ;
#46761=CARTESIAN_POINT('',(18.7,6.35,42.5)) ;
#46762=CARTESIAN_POINT('Origin',(18.7,6.35,42.6)) ;
#46763=CARTESIAN_POINT('',(18.7,6.8,42.6)) ;
#46764=CARTESIAN_POINT('Origin',(18.8,6.8,42.6)) ;
#46765=CARTESIAN_POINT('',(18.9,6.8,42.6)) ;
#46766=CARTESIAN_POINT('Origin',(18.9,6.35,42.6)) ;
#46767=CARTESIAN_POINT('Origin',(17.9,6.8,42.6)) ;
#46768=CARTESIAN_POINT('',(17.8,6.8,42.5)) ;
#46769=CARTESIAN_POINT('',(17.8,6.8,42.6)) ;
#46770=CARTESIAN_POINT('',(18.,6.8,42.5)) ;
#46771=CARTESIAN_POINT('',(17.9,6.8,42.5)) ;
#46772=CARTESIAN_POINT('',(18.,6.8,42.6)) ;
#46773=CARTESIAN_POINT('Origin',(18.,6.35,42.6)) ;
#46774=CARTESIAN_POINT('',(18.,6.35,42.5)) ;
#46775=CARTESIAN_POINT('Origin',(17.9,6.35,42.5)) ;
#46776=CARTESIAN_POINT('',(17.8,6.35,42.5)) ;
#46777=CARTESIAN_POINT('Origin',(17.8,6.35,42.6)) ;
#46778=CARTESIAN_POINT('Origin',(17.,6.35,42.5)) ;
#46779=CARTESIAN_POINT('',(17.1,6.8,42.5)) ;
#46780=CARTESIAN_POINT('',(17.1,6.35,42.5)) ;
#46781=CARTESIAN_POINT('',(16.9,6.8,42.5)) ;
#46782=CARTESIAN_POINT('',(17.,6.8,42.5)) ;
#46783=CARTESIAN_POINT('',(16.9,6.35,42.5)) ;
#46784=CARTESIAN_POINT('Origin',(16.9,6.35,42.6)) ;
#46785=CARTESIAN_POINT('',(16.9,6.8,42.6)) ;
#46786=CARTESIAN_POINT('Origin',(17.,6.8,42.6)) ;
#46787=CARTESIAN_POINT('',(17.1,6.8,42.6)) ;
#46788=CARTESIAN_POINT('Origin',(17.1,6.35,42.6)) ;
#46789=CARTESIAN_POINT('Origin',(20.5,6.6,42.4)) ;
#46790=CARTESIAN_POINT('',(24.5,7.2,42.4)) ;
#46791=CARTESIAN_POINT('',(24.5,6.6,42.4)) ;
#46792=CARTESIAN_POINT('',(16.5,7.2,42.4)) ;
#46793=CARTESIAN_POINT('',(16.5,6.6,42.4)) ;
#46794=CARTESIAN_POINT('',(20.5,7.2,42.4)) ;
#46795=CARTESIAN_POINT('Origin',(16.5,6.6,42.5)) ;
#46796=CARTESIAN_POINT('',(16.5,7.2,42.5)) ;
#46797=CARTESIAN_POINT('Origin',(20.5,7.2,42.5)) ;
#46798=CARTESIAN_POINT('',(24.5,7.2,42.5)) ;
#46799=CARTESIAN_POINT('Origin',(24.5,6.6,42.5)) ;
#50361=UNCERTAINTY_MEASURE_WITH_UNIT(LENGTH_MEASURE(0.001),#50441,
'DISTANCE_ACCURACY_VALUE',
'Maximum model space distance between geometric entities at asserted c
onnectivities') ;
#50387=UNCERTAINTY_MEASURE_WITH_UNIT(LENGTH_MEASURE(0.001),#50441,
'DISTANCE_ACCURACY_VALUE',
'Maximum model space distance between geometric entities at asserted c
onnectivities') ;
#50414=(
GEOMETRIC_REPRESENTATION_CONTEXT(3)
GLOBAL_UNCERTAINTY_ASSIGNED_CONTEXT((#50361))
GLOBAL_UNIT_ASSIGNED_CONTEXT((#50441,#50443,#50444))
REPRESENTATION_CONTEXT('','3D')
) ;
#50440=(
GEOMETRIC_REPRESENTATION_CONTEXT(3)
GLOBAL_UNCERTAINTY_ASSIGNED_CONTEXT((#50387))
GLOBAL_UNIT_ASSIGNED_CONTEXT((#50441,#50443,#50444))
REPRESENTATION_CONTEXT('','3D')
) ;
#50441=(
LENGTH_UNIT()
NAMED_UNIT(*)
SI_UNIT(.CENTI.,.METRE.)
) ;
#50443=(
NAMED_UNIT(*)
PLANE_ANGLE_UNIT()
SI_UNIT($,.RADIAN.)
) ;
#50444=(
NAMED_UNIT(*)
SI_UNIT($,.STERADIAN.)
SOLID_ANGLE_UNIT()
) ;
#50471=SHAPE_DEFINITION_REPRESENTATION(#50547,#50645) ;
#50547=PRODUCT_DEFINITION_SHAPE('',$,#50698) ;
#50645=SHAPE_REPRESENTATION('',(#30765),#50414) ;
#50671=PRODUCT_DEFINITION_CONTEXT('part definition',#50829,'design') ;
#50698=PRODUCT_DEFINITION('FLOW_RATE_SCALE_STRIP',
'FLOW_RATE_SCALE_STRIP',#50750,#50671) ;
#50750=PRODUCT_DEFINITION_FORMATION('',$,#50857) ;
#50829=APPLICATION_CONTEXT(
'Core Data for Automotive Mechanical Design Process') ;
#50830=PRODUCT_CONTEXT('part definition',#50829,'mechanical') ;
#50857=PRODUCT('FLOW_RATE_SCALE_STRIP','FLOW_RATE_SCALE_STRIP',$,(#50830)) ;
#50886=PRESENTATION_STYLE_ASSIGNMENT((#50893)) ;
#50893=SURFACE_STYLE_USAGE(.BOTH.,#50900) ;
#50900=SURFACE_SIDE_STYLE('',(#50907)) ;
#50907=SURFACE_STYLE_FILL_AREA(#50914) ;
#50914=FILL_AREA_STYLE('Aluminum - Satin',(#50921)) ;
#50921=FILL_AREA_STYLE_COLOUR('Aluminum - Satin',#50928) ;
#50928=COLOUR_RGB('Aluminum - Satin', 0.09019608, 0.27058824, 0.51372549) ;
ENDSEC;
END-ISO-10303-21;
